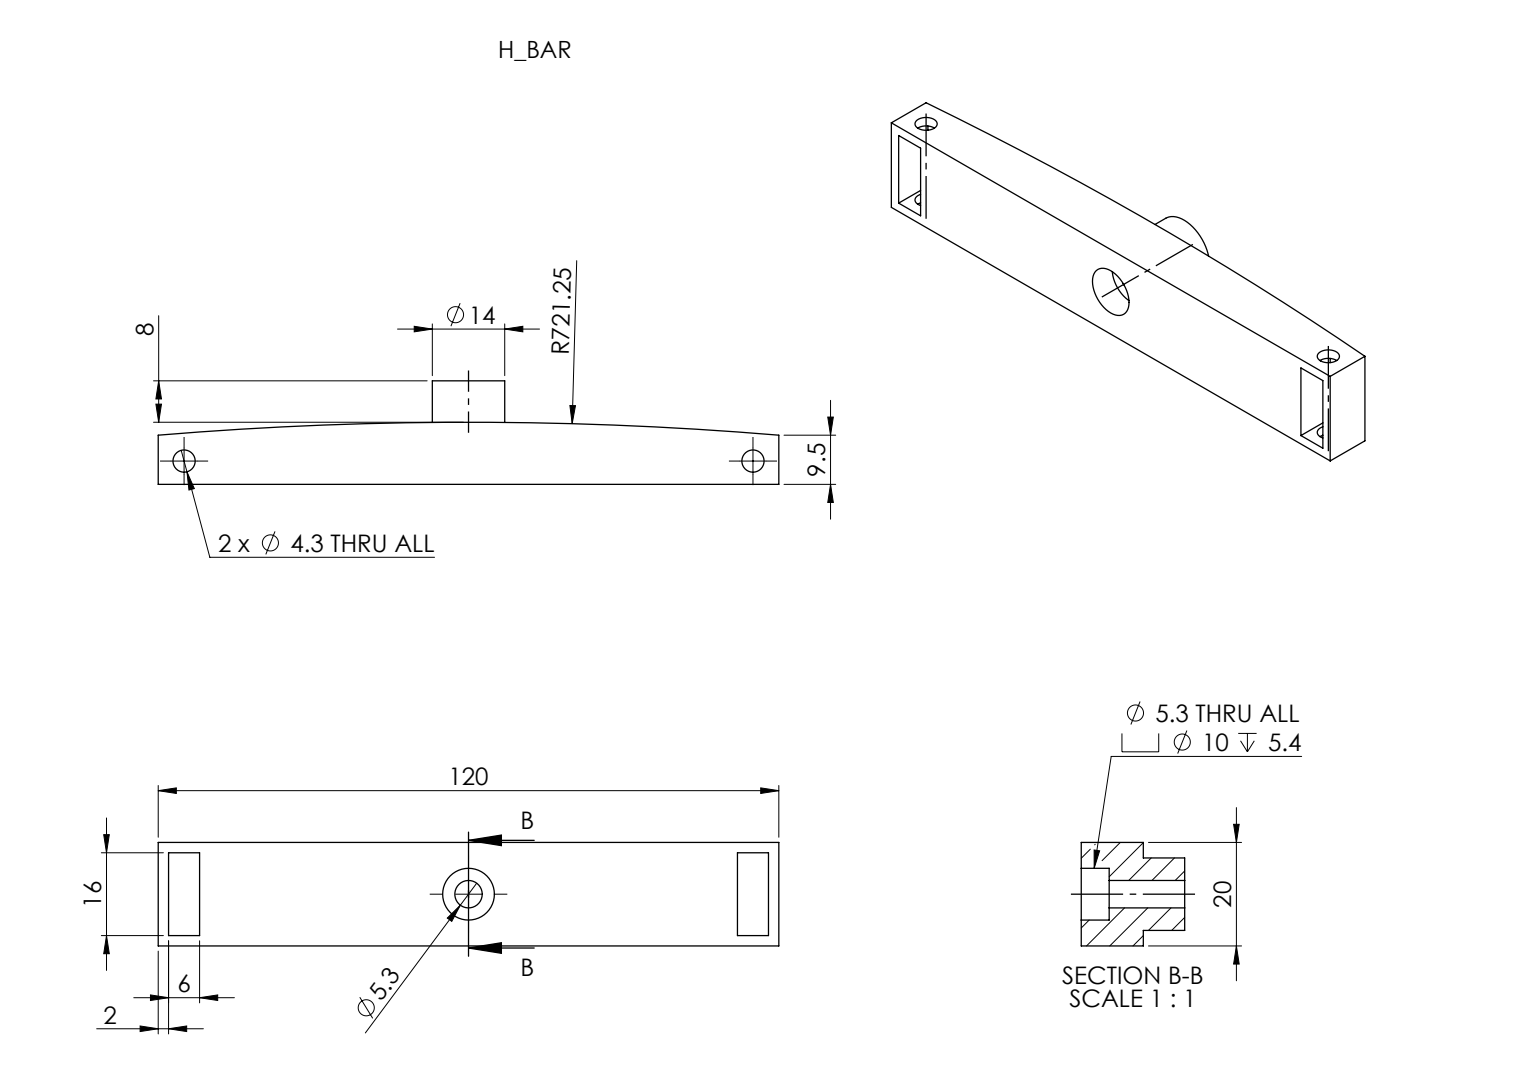
ISO-10303-21;
HEADER;
FILE_DESCRIPTION (('STEP AP214'),
    '1' );
FILE_NAME ('H_bar.step',
    '2026-10-08T12:12:07',
    ( '' ),
    ( '' ),
    'SwSTEP 2.0',
    'SolidWorks 2026',
    '' );
FILE_SCHEMA (( 'AUTOMOTIVE_DESIGN' ));
ENDSEC;

DATA;
#33=EDGE_CURVE ( 'NONE', #5370, #4266, #4037, .T. ) ;
#35=DIRECTION ( 'NONE',  ( 0.000000000000000000, -0.000000000000000000, -1.000000000000000000 ) ) ;
#36=CARTESIAN_POINT ( 'NONE',  ( -54.99999999999990052, 7.999999999999996447, 17.64999999999876579 ) ) ;
#37=CARTESIAN_POINT ( 'NONE',  ( 2.649999999999999023, 0.000000000000000000, 20.00000000000000355 ) ) ;
#43=ORIENTED_EDGE ( 'NONE', *, *, #111, .F. ) ;
#49=ORIENTED_EDGE ( 'NONE', *, *, #6995, .T. ) ;
#50=EDGE_CURVE ( 'NONE', #5044, #7574, #6013, .T. ) ;
#62=FACE_OUTER_BOUND ( 'NONE', #6300, .T. ) ;
#67=FACE_OUTER_BOUND ( 'NONE', #4002, .T. ) ;
#88=EDGE_CURVE ( 'NONE', #1891, #7622, #3368, .T. ) ;
#95=DIRECTION ( 'NONE',  ( -1.000000000000000000, 0.000000000000000000, 7.304098846218136639E-16 ) ) ;
#98=FACE_OUTER_BOUND ( 'NONE', #4834, .T. ) ;
#99=VECTOR ( 'NONE', #2043, 1000.000000000000000 ) ;
#103=CARTESIAN_POINT ( 'NONE',  ( 57.99999999999999289, 7.999999999999996447, 11.99999999999998934 ) ) ;
#111=EDGE_CURVE ( 'NONE', #2701, #7610, #4070, .T. ) ;
#120=VECTOR ( 'NONE', #1322, 1000.000000000000000 ) ;
#125=DIRECTION ( 'NONE',  ( 0.000000000000000000, 0.000000000000000000, 1.000000000000000000 ) ) ;
#130=AXIS2_PLACEMENT_3D ( 'NONE', #7551, #5648, #7466 ) ;
#132=ORIENTED_EDGE ( 'NONE', *, *, #3473, .T. ) ;
#142=CARTESIAN_POINT ( 'NONE',  ( 60.00000000000000711, 10.00000000000000000, 19.99999999999998224 ) ) ;
#147=EDGE_CURVE ( 'NONE', #4940, #6473, #5403, .T. ) ;
#149=ORIENTED_EDGE ( 'NONE', *, *, #1842, .T. ) ;
#156=CIRCLE ( 'NONE', #5095, 721.2499999999977263 ) ;
#162=ORIENTED_EDGE ( 'NONE', *, *, #3354, .T. ) ;
#179=EDGE_CURVE ( 'NONE', #2593, #4900, #5449, .T. ) ;
#188=LINE ( 'NONE', #4647, #2150 ) ;
#193=CARTESIAN_POINT ( 'NONE',  ( 52.00000000000000000, 7.999999999999996447, 19.99999999999998934 ) ) ;
#203=CARTESIAN_POINT ( 'NONE',  ( 1.817638007539982281, -6.775366854781982084, 8.002150721412645495 ) ) ;
#239=CIRCLE ( 'NONE', #4755, 2.650000000000010125 ) ;
#240=ORIENTED_EDGE ( 'NONE', *, *, #3379, .F. ) ;
#247=CARTESIAN_POINT ( 'NONE',  ( 6.063862694340463655, -3.504607373393594294, 8.025483085394268912 ) ) ;
#249=AXIS2_PLACEMENT_3D ( 'NONE', #6671, #347, #6580 ) ;
#253=EDGE_CURVE ( 'NONE', #6951, #2122, #5644, .T. ) ;
#262=DIRECTION ( 'NONE',  ( 0.000000000000000000, 0.000000000000000000, -1.000000000000000000 ) ) ;
#284=ORIENTED_EDGE ( 'NONE', *, *, #776, .T. ) ;
#286=CARTESIAN_POINT ( 'NONE',  ( 6.775412730438223896, -1.817364742217071338, 8.031819226609355766 ) ) ;
#289=PRODUCT_DEFINITION_FORMATION_WITH_SPECIFIED_SOURCE ( 'ANY', '', #1201, .NOT_KNOWN. ) ;
#292=EDGE_CURVE ( 'NONE', #5760, #2794, #1287, .T. ) ;
#313=CIRCLE ( 'NONE', #3509, 7.000000000000000000 ) ;
#315=EDGE_LOOP ( 'NONE', ( #5277, #4331 ) ) ;
#323=ORIENTED_EDGE ( 'NONE', *, *, #6415, .F. ) ;
#329=EDGE_CURVE ( 'NONE', #4266, #3008, #313, .T. ) ;
#335=SURFACE_STYLE_USAGE ( .BOTH. , #876 ) ;
#337=CARTESIAN_POINT ( 'NONE',  ( 55.00000000000000000, -8.000000000000001776, 17.64999999999999858 ) ) ;
#347=DIRECTION ( 'NONE',  ( -0.000000000000000000, 1.000000000000000000, -0.000000000000000000 ) ) ;
#350=LINE ( 'NONE', #2279, #863 ) ;
#357=DIRECTION ( 'NONE',  ( 0.000000000000000000, 0.000000000000000000, 1.000000000000000000 ) ) ;
#361=CARTESIAN_POINT ( 'NONE',  ( -58.00000000000006395, -8.000000000000003553, 19.99999999999998934 ) ) ;
#364=EDGE_LOOP ( 'NONE', ( #6417, #7648 ) ) ;
#369=CARTESIAN_POINT ( 'NONE',  ( -60.00000000000000000, 10.00000000000000000, 20.00000000000000355 ) ) ;
#370=CARTESIAN_POINT ( 'NONE',  ( -3.469446951953613006E-15, 0.000000000000000000, 20.00000000000000355 ) ) ;
#382=CARTESIAN_POINT ( 'NONE',  ( -6.821151181492251858, -1.588688383954758754, 8.032254533892484005 ) ) ;
#385=DIRECTION ( 'NONE',  ( -1.000000000000000000, 0.000000000000000000, -0.000000000000000000 ) ) ;
#398=EDGE_CURVE ( 'NONE', #2960, #580, #3789, .T. ) ;
#399=CARTESIAN_POINT ( 'NONE',  ( -3.469446951953613006E-15, 0.000000000000000000, 14.60000000000000142 ) ) ;
#400=EDGE_CURVE ( 'NONE', #3913, #5044, #2617, .T. ) ;
#417=VECTOR ( 'NONE', #2244, 1000.000000000000000 ) ;
#426=CARTESIAN_POINT ( 'NONE',  ( -7.000000000000002665, -0.4626139278909737751, 8.033969604113735841 ) ) ;
#427=CARTESIAN_POINT ( 'NONE',  ( 5.563937487951679195, 4.272621587589405578, 8.021415735625629040 ) ) ;
#431=FILL_AREA_STYLE ('',( #5077 ) ) ;
#439=CARTESIAN_POINT ( 'NONE',  ( 52.00000000000000000, 7.999999999999996447, 19.99999999999998934 ) ) ;
#454=ADVANCED_FACE ( 'NONE', ( #5886, #6459 ), #5961, .F. ) ;
#458=CYLINDRICAL_SURFACE ( 'NONE', #3417, 4.999999999999993783 ) ;
#466=DIRECTION ( 'NONE',  ( 0.000000000000000000, -1.000000000000000000, 0.000000000000000000 ) ) ;
#470=CARTESIAN_POINT ( 'NONE',  ( 4.263933714126141972, 5.556256305342602175, 8.012582018583044530 ) ) ;
#471=VERTEX_POINT ( 'NONE', #2181 ) ;
#481=CARTESIAN_POINT ( 'NONE',  ( 9.020562075079396891E-14, 10.00000000000000000, 8.000000000000007105 ) ) ;
#485=EDGE_CURVE ( 'NONE', #5247, #2461, #7128, .T. ) ;
#492=ORIENTED_EDGE ( 'NONE', *, *, #3666, .F. ) ;
#496=DIRECTION ( 'NONE',  ( -0.000000000000000000, 1.000000000000000000, -0.000000000000000000 ) ) ;
#497=CARTESIAN_POINT ( 'NONE',  ( -58.00000000000006395, -8.000000000000003553, 11.99999999999998934 ) ) ;
#503=DIRECTION ( 'NONE',  ( -0.000000000000000000, -0.000000000000000000, 1.000000000000000000 ) ) ;
#533=ORIENTED_EDGE ( 'NONE', *, *, #8046, .T. ) ;
#537=DIRECTION ( 'NONE',  ( 0.000000000000000000, -1.000000000000000000, 0.000000000000000000 ) ) ;
#542=CIRCLE ( 'NONE', #6772, 2.149999999999995470 ) ;
#545=EDGE_LOOP ( 'NONE', ( #3135, #132, #1061, #2329, #6550 ) ) ;
#562=AXIS2_PLACEMENT_3D ( 'NONE', #5807, #845, #6662 ) ;
#579=EDGE_LOOP ( 'NONE', ( #6634, #3876, #4463, #3342 ) ) ;
#580=VERTEX_POINT ( 'NONE', #4679 ) ;
#585=FACE_OUTER_BOUND ( 'NONE', #4794, .T. ) ;
#615=LINE ( 'NONE', #8136, #2509 ) ;
#622=ORIENTED_EDGE ( 'NONE', *, *, #7733, .F. ) ;
#625=ORIENTED_EDGE ( 'NONE', *, *, #147, .F. ) ;
#627=CARTESIAN_POINT ( 'NONE',  ( -52.00000000000006395, 7.999999999999996447, 19.99999999999998934 ) ) ;
#628=CARTESIAN_POINT ( 'NONE',  ( -3.469446951953613006E-15, 0.000000000000000000, 1.040834085586084257E-14 ) ) ;
#630=ORIENTED_EDGE ( 'NONE', *, *, #4013, .F. ) ;
#639=CARTESIAN_POINT ( 'NONE',  ( -3.469446951953613006E-15, 0.000000000000000000, 20.00000000000000355 ) ) ;
#660=DIRECTION ( 'NONE',  ( -0.000000000000000000, 1.000000000000000000, -0.000000000000000000 ) ) ;
#661=VECTOR ( 'NONE', #6389, 1000.000000000000000 ) ;
#664=CARTESIAN_POINT ( 'NONE',  ( -54.99999999999990052, 10.00000000000000000, 13.34999999999877218 ) ) ;
#674=ORIENTED_EDGE ( 'NONE', *, *, #5759, .F. ) ;
#692=PLANE ( 'NONE',  #3596 ) ;
#698=CARTESIAN_POINT ( 'NONE',  ( -2.649999999999998579, 3.245314017740484976E-16, 1.040834085586084257E-14 ) ) ;
#710=DIRECTION ( 'NONE',  ( 0.000000000000000000, 0.000000000000000000, -1.000000000000000000 ) ) ;
#718=EDGE_CURVE ( 'NONE', #6876, #5247, #3796, .T. ) ;
#725=EDGE_CURVE ( 'NONE', #4369, #7382, #3169, .T. ) ;
#729=FACE_OUTER_BOUND ( 'NONE', #7926, .T. ) ;
#736=ORIENTED_EDGE ( 'NONE', *, *, #147, .T. ) ;
#737=ORIENTED_EDGE ( 'NONE', *, *, #4756, .F. ) ;
#745=CARTESIAN_POINT ( 'NONE',  ( -54.99999999999990052, 7.999999999999996447, 15.49999999999877254 ) ) ;
#746=ORIENTED_EDGE ( 'NONE', *, *, #292, .T. ) ;
#747=ORIENTED_EDGE ( 'NONE', *, *, #7686, .F. ) ;
#751=DIRECTION ( 'NONE',  ( -0.000000000000000000, 1.000000000000000000, -0.000000000000000000 ) ) ;
#755=AXIS2_PLACEMENT_3D ( 'NONE', #7446, #2992, #997 ) ;
#756=CIRCLE ( 'NONE', #6069, 2.149999999999995470 ) ;
#759=DIRECTION ( 'NONE',  ( 0.000000000000000000, 0.000000000000000000, 1.000000000000000000 ) ) ;
#762=LINE ( 'NONE', #7672, #2341 ) ;
#764=ORIENTED_EDGE ( 'NONE', *, *, #3354, .F. ) ;
#765=DIRECTION ( 'NONE',  ( -0.000000000000000000, -0.000000000000000000, 1.000000000000000000 ) ) ;
#769=FACE_BOUND ( 'NONE', #5362, .T. ) ;
#775=VECTOR ( 'NONE', #2784, 1000.000000000000000 ) ;
#776=EDGE_CURVE ( 'NONE', #7532, #6647, #3721, .T. ) ;
#783=EDGE_LOOP ( 'NONE', ( #2328, #2669, #3779, #4427 ) ) ;
#796=CARTESIAN_POINT ( 'NONE',  ( -58.00000000000006395, -8.000000000000003553, 11.99999999999998934 ) ) ;
#797=EDGE_CURVE ( 'NONE', #3149, #2513, #8163, .T. ) ;
#805=CARTESIAN_POINT ( 'NONE',  ( 60.00000000000000711, 10.00000000000000000, 19.99999999999998224 ) ) ;
#812=LINE ( 'NONE', #1377, #1681 ) ;
#813=LINE ( 'NONE', #4683, #1169 ) ;
#816=CARTESIAN_POINT ( 'NONE',  ( 9.020562075079396891E-14, 10.00000000000000000, 729.2499999999977263 ) ) ;
#831=CARTESIAN_POINT ( 'NONE',  ( -3.469446951953613006E-15, 0.000000000000000000, 20.00000000000000355 ) ) ;
#833=( GEOMETRIC_REPRESENTATION_CONTEXT ( 3 ) GLOBAL_UNCERTAINTY_ASSIGNED_CONTEXT ( ( #1043 ) ) GLOBAL_UNIT_ASSIGNED_CONTEXT ( ( #7363, #5472, #1683 ) ) REPRESENTATION_CONTEXT ( 'NONE', 'WORKASPACE' ) );
#835=CARTESIAN_POINT ( 'NONE',  ( 60.00000000000000711, 10.00000000000000000, 19.99999999999998224 ) ) ;
#836=ADVANCED_FACE ( 'NONE', ( #2976 ), #4986, .T. ) ;
#838=EDGE_CURVE ( 'NONE', #5760, #2420, #5577, .T. ) ;
#841=DIRECTION ( 'NONE',  ( 0.000000000000000000, 0.000000000000000000, 1.000000000000000000 ) ) ;
#845=DIRECTION ( 'NONE',  ( -0.000000000000000000, -0.000000000000000000, 1.000000000000000000 ) ) ;
#863=VECTOR ( 'NONE', #7874, 1000.000000000000000 ) ;
#864=ORIENTED_EDGE ( 'NONE', *, *, #4147, .T. ) ;
#865=DIRECTION ( 'NONE',  ( 0.000000000000000000, -1.000000000000000000, 0.000000000000000000 ) ) ;
#870=AXIS2_PLACEMENT_3D ( 'NONE', #103, #5737, #2689 ) ;
#873=DIRECTION ( 'NONE',  ( 0.000000000000000000, 0.000000000000000000, 1.000000000000000000 ) ) ;
#875=B_SPLINE_CURVE_WITH_KNOTS ( 'NONE', 3,
 ( #6650, #6025, #2207, #203, #2749, #5292, #3377, #4666, #2168, #2092, #7318, #914, #2714, #5986, #247, #3500, #4704, #2797, #286, #4791, #957, #4623 ),
 .UNSPECIFIED., .F., .F.,
 ( 4, 2, 2, 2, 2, 2, 2, 2, 2, 2, 4 ),
 ( 0.01094514227676123691, 0.01231266565124741405, 0.01368018902573359119, 0.01436395071297667803, 0.01504771240021976486, 0.01641523577470593853, 0.01778275914919211220, 0.01846652083643519904, 0.01915028252367827893, 0.02051780589816445260, 0.02188532927265061934 ),
 .UNSPECIFIED. ) ;
#876=SURFACE_SIDE_STYLE ('',( #6615 ) ) ;
#882=EDGE_LOOP ( 'NONE', ( #6137, #7790, #7495, #985 ) ) ;
#885=DIRECTION ( 'NONE',  ( 0.000000000000000000, 0.000000000000000000, -1.000000000000000000 ) ) ;
#895=EDGE_LOOP ( 'NONE', ( #149, #7973 ) ) ;
#908=ORIENTED_EDGE ( 'NONE', *, *, #1318, .T. ) ;
#914=CARTESIAN_POINT ( 'NONE',  ( 5.276116561136752203, -4.623420808406671689, 8.019224293709841689 ) ) ;
#923=CARTESIAN_POINT ( 'NONE',  ( 55.00000000000000000, 7.999999999999996447, 15.50000000000000355 ) ) ;
#927=APPLICATION_CONTEXT ( 'automotive_design' ) ;
#929=DIRECTION ( 'NONE',  ( 1.000000000000000000, 0.000000000000000000, -1.734723475976807094E-16 ) ) ;
#938=CARTESIAN_POINT ( 'NONE',  ( 57.99999999999999289, 7.999999999999996447, 11.99999999999998934 ) ) ;
#943=ORIENTED_EDGE ( 'NONE', *, *, #5994, .T. ) ;
#945=EDGE_CURVE ( 'NONE', #2445, #7873, #4769, .T. ) ;
#947=CARTESIAN_POINT ( 'NONE',  ( -54.99999999999990052, -8.000000000000001776, 13.34999999999877573 ) ) ;
#957=CARTESIAN_POINT ( 'NONE',  ( 7.000000000000000000, -0.4567577452614210998, 8.033969604113657681 ) ) ;
#963=ADVANCED_FACE ( 'NONE', ( #4403 ), #7637, .F. ) ;
#967=PLANE ( 'NONE',  #3326 ) ;
#980=LINE ( 'NONE', #938, #4549 ) ;
#984=ORIENTED_EDGE ( 'NONE', *, *, #6326, .T. ) ;
#985=ORIENTED_EDGE ( 'NONE', *, *, #7008, .T. ) ;
#988=CARTESIAN_POINT ( 'NONE',  ( 55.00000000000000000, 7.999999999999996447, 17.64999999999999858 ) ) ;
#997=DIRECTION ( 'NONE',  ( 0.000000000000000000, 0.000000000000000000, -1.000000000000000000 ) ) ;
#999=ORIENTED_EDGE ( 'NONE', *, *, #1723, .T. ) ;
#1007=CIRCLE ( 'NONE', #3821, 2.149999999999992362 ) ;
#1008=ADVANCED_FACE ( 'NONE', ( #3156, #7748 ), #692, .F. ) ;
#1009=EDGE_CURVE ( 'NONE', #2513, #7631, #542, .T. ) ;
#1011=FACE_OUTER_BOUND ( 'NONE', #3128, .T. ) ;
#1012=ORIENTED_EDGE ( 'NONE', *, *, #945, .F. ) ;
#1020=ORIENTED_EDGE ( 'NONE', *, *, #4149, .F. ) ;
#1022=ORIENTED_EDGE ( 'NONE', *, *, #3595, .F. ) ;
#1032=AXIS2_PLACEMENT_3D ( 'NONE', #745, #2051, #5285 ) ;
#1039=CARTESIAN_POINT ( 'NONE',  ( 0.000000000000000000, 0.000000000000000000, 0.000000000000000000 ) ) ;
#1043=UNCERTAINTY_MEASURE_WITH_UNIT (LENGTH_MEASURE( 1.000000000000000082E-05 ), #7363, 'distance_accuracy_value', 'NONE');
#1057=FACE_OUTER_BOUND ( 'NONE', #7251, .T. ) ;
#1059=ORIENTED_EDGE ( 'NONE', *, *, #7565, .F. ) ;
#1061=ORIENTED_EDGE ( 'NONE', *, *, #2412, .T. ) ;
#1068=EDGE_LOOP ( 'NONE', ( #6038, #2674, #6851, #8178 ) ) ;
#1071=ORIENTED_EDGE ( 'NONE', *, *, #8119, .F. ) ;
#1083=CARTESIAN_POINT ( 'NONE',  ( -60.00000000000000000, -10.00000000000000000, 10.50000000000000000 ) ) ;
#1091=DIRECTION ( 'NONE',  ( -0.000000000000000000, 1.000000000000000000, -0.000000000000000000 ) ) ;
#1101=EDGE_LOOP ( 'NONE', ( #4231, #1354, #3513, #6258 ) ) ;
#1107=DIRECTION ( 'NONE',  ( 0.000000000000000000, 1.000000000000000000, -0.000000000000000000 ) ) ;
#1116=CARTESIAN_POINT ( 'NONE',  ( -1.809537700406288696, 6.765955536481263799, 8.002236580937831079 ) ) ;
#1127=LINE ( 'NONE', #6150, #6601 ) ;
#1131=CYLINDRICAL_SURFACE ( 'NONE', #4595, 4.999999999999993783 ) ;
#1152=PLANE ( 'NONE',  #2816 ) ;
#1169=VECTOR ( 'NONE', #6434, 1000.000000000000000 ) ;
#1175=CIRCLE ( 'NONE', #5826, 2.649999999999995026 ) ;
#1189=EDGE_LOOP ( 'NONE', ( #4336, #622, #5682, #3680 ) ) ;
#1197=VECTOR ( 'NONE', #3237, 1000.000000000000000 ) ;
#1201=PRODUCT ( 'H_bar', 'H_bar', '', ( #3408 ) ) ;
#1205=CARTESIAN_POINT ( 'NONE',  ( 55.00000000000000000, -8.000000000000001776, 13.35000000000000853 ) ) ;
#1209=LINE ( 'NONE', #37, #3965 ) ;
#1242=CARTESIAN_POINT ( 'NONE',  ( -54.99999999999990052, -8.000000000000001776, 15.49999999999877254 ) ) ;
#1275=ORIENTED_EDGE ( 'NONE', *, *, #838, .F. ) ;
#1280=CARTESIAN_POINT ( 'NONE',  ( -60.00000000000000000, -10.00000000000000000, 20.00000000000000355 ) ) ;
#1282=EDGE_CURVE ( 'NONE', #5386, #4369, #4820, .T. ) ;
#1287=LINE ( 'NONE', #5085, #2062 ) ;
#1307=ORIENTED_EDGE ( 'NONE', *, *, #1889, .T. ) ;
#1308=ORIENTED_EDGE ( 'NONE', *, *, #400, .T. ) ;
#1313=CARTESIAN_POINT ( 'NONE',  ( -0.4566803630309465567, -7.000000000000006217, 8.000000000000042633 ) ) ;
#1315=ADVANCED_FACE ( 'NONE', ( #4557 ), #3144, .T. ) ;
#1318=EDGE_CURVE ( 'NONE', #6647, #5567, #5729, .T. ) ;
#1320=DIRECTION ( 'NONE',  ( -0.000000000000000000, 1.000000000000000000, -0.000000000000000000 ) ) ;
#1322=DIRECTION ( 'NONE',  ( -7.304098846218136639E-16, 0.000000000000000000, -1.000000000000000000 ) ) ;
#1331=ORIENTED_EDGE ( 'NONE', *, *, #179, .T. ) ;
#1337=CARTESIAN_POINT ( 'NONE',  ( 9.020562075079396891E-14, 10.00000000000000000, 729.2499999999977263 ) ) ;
#1342=VECTOR ( 'NONE', #7696, 1000.000000000000000 ) ;
#1354=ORIENTED_EDGE ( 'NONE', *, *, #3875, .F. ) ;
#1361=DIRECTION ( 'NONE',  ( -0.000000000000000000, -0.000000000000000000, 1.000000000000000000 ) ) ;
#1368=SHAPE_REPRESENTATION ( 'H_bar', ( #1587 ), #2170 ) ;
#1377=CARTESIAN_POINT ( 'NONE',  ( 52.00000000000000000, 7.999999999999996447, 11.99999999999998934 ) ) ;
#1381=ORIENTED_EDGE ( 'NONE', *, *, #725, .F. ) ;
#1389=CARTESIAN_POINT ( 'NONE',  ( -54.99999999999990052, -8.000000000000001776, 17.64999999999876579 ) ) ;
#1393=ORIENTED_EDGE ( 'NONE', *, *, #6516, .T. ) ;
#1399=CARTESIAN_POINT ( 'NONE',  ( -3.094755790304997145, -6.282913975126477979, 8.006611220574070487 ) ) ;
#1400=VECTOR ( 'NONE', #765, 1000.000000000000000 ) ;
#1421=AXIS2_PLACEMENT_3D ( 'NONE', #4138, #4718, #1488 ) ;
#1423=CARTESIAN_POINT ( 'NONE',  ( 52.00000000000000000, -8.000000000000003553, 11.99999999999998934 ) ) ;
#1430=EDGE_LOOP ( 'NONE', ( #2699, #674, #6368, #3754 ) ) ;
#1445=DIRECTION ( 'NONE',  ( -0.000000000000000000, 1.000000000000000000, -0.000000000000000000 ) ) ;
#1448=CARTESIAN_POINT ( 'NONE',  ( 2.650000000000006573, 0.000000000000000000, 14.60000000000000142 ) ) ;
#1461=VERTEX_POINT ( 'NONE', #835 ) ;
#1482=CYLINDRICAL_SURFACE ( 'NONE', #7579, 2.149999999999995470 ) ;
#1488=DIRECTION ( 'NONE',  ( -1.000000000000000000, 0.000000000000000000, 0.000000000000000000 ) ) ;
#1503=ORIENTED_EDGE ( 'NONE', *, *, #4756, .T. ) ;
#1516=( NAMED_UNIT ( * ) SI_UNIT ( $, .STERADIAN. ) SOLID_ANGLE_UNIT ( ) );
#1518=CARTESIAN_POINT ( 'NONE',  ( 6.764948177723724143, 1.813303243961031264, 8.031723462610594666 ) ) ;
#1544=FACE_BOUND ( 'NONE', #3563, .T. ) ;
#1551=FILL_AREA_STYLE ('',( #6745 ) ) ;
#1557=STYLED_ITEM ( 'NONE', ( #1912 ), #6918 ) ;
#1562=DIRECTION ( 'NONE',  ( -7.304098846218136639E-16, 0.000000000000000000, -1.000000000000000000 ) ) ;
#1565=CARTESIAN_POINT ( 'NONE',  ( 55.00000000000000000, 10.00000000000000000, 17.65000000000000213 ) ) ;
#1581=CARTESIAN_POINT ( 'NONE',  ( -5.560873836092222078, 4.276402017733387240, 8.021392354376160938 ) ) ;
#1585=ADVANCED_FACE ( 'NONE', ( #4332 ), #1131, .F. ) ;
#1587=AXIS2_PLACEMENT_3D ( 'NONE', #3942, #5152, #6454 ) ;
#1588=ORIENTED_EDGE ( 'NONE', *, *, #3229, .F. ) ;
#1611=LINE ( 'NONE', #2935, #3551 ) ;
#1612=CARTESIAN_POINT ( 'NONE',  ( 55.00000000000000000, 7.999999999999996447, 13.35000000000000853 ) ) ;
#1613=LINE ( 'NONE', #7372, #4745 ) ;
#1615=CARTESIAN_POINT ( 'NONE',  ( -52.00000000000006395, -8.000000000000003553, 11.99999999999998934 ) ) ;
#1625=CARTESIAN_POINT ( 'NONE',  ( -7.000000000000000000, 0.4621588634683668206, 8.033969604113732288 ) ) ;
#1628=AXIS2_PLACEMENT_3D ( 'NONE', #2103, #4640, #7863 ) ;
#1638=DIRECTION ( 'NONE',  ( -0.000000000000000000, -1.000000000000000000, -0.000000000000000000 ) ) ;
#1642=MECHANICAL_DESIGN_GEOMETRIC_PRESENTATION_REPRESENTATION('',(#5233),#833);
#1644=DIRECTION ( 'NONE',  ( -0.000000000000000000, 1.000000000000000000, -0.000000000000000000 ) ) ;
#1645=CARTESIAN_POINT ( 'NONE',  ( -6.290416253262643309, -3.105047250628316213, 8.027410178832276699 ) ) ;
#1657=EDGE_LOOP ( 'NONE', ( #1071, #737 ) ) ;
#1660=ORIENTED_EDGE ( 'NONE', *, *, #5235, .T. ) ;
#1669=ORIENTED_EDGE ( 'NONE', *, *, #3413, .F. ) ;
#1681=VECTOR ( 'NONE', #5239, 1000.000000000000000 ) ;
#1682=AXIS2_PLACEMENT_3D ( 'NONE', #4853, #2353, #4946 ) ;
#1683=( NAMED_UNIT ( * ) SI_UNIT ( $, .STERADIAN. ) SOLID_ANGLE_UNIT ( ) );
#1685=CARTESIAN_POINT ( 'NONE',  ( 6.282784822387311507, 3.095002094042488050, 8.027357021320174368 ) ) ;
#1690=DIRECTION ( 'NONE',  ( -0.000000000000000000, -1.000000000000000000, -0.000000000000000000 ) ) ;
#1700=VECTOR ( 'NONE', #5315, 1000.000000000000000 ) ;
#1723=EDGE_CURVE ( 'NONE', #7610, #1891, #350, .T. ) ;
#1727=VERTEX_POINT ( 'NONE', #2899 ) ;
#1743=DIRECTION ( 'NONE',  ( 1.000000000000000000, 0.000000000000000000, -1.734723475976807094E-16 ) ) ;
#1748=ORIENTED_EDGE ( 'NONE', *, *, #3669, .T. ) ;
#1749=ORIENTED_EDGE ( 'NONE', *, *, #2036, .T. ) ;
#1759=ORIENTED_EDGE ( 'NONE', *, *, #8046, .F. ) ;
#1765=CIRCLE ( 'NONE', #3887, 4.999999999999993783 ) ;
#1771=CARTESIAN_POINT ( 'NONE',  ( -54.99999999999990052, 10.00000000000000000, 15.49999999999877254 ) ) ;
#1774=CARTESIAN_POINT ( 'NONE',  ( 9.020562070449730010E-14, 7.000000000000000000, 8.000000000000058620 ) ) ;
#1780=DIRECTION ( 'NONE',  ( 0.000000000000000000, 1.000000000000000000, -0.000000000000000000 ) ) ;
#1787=ORIENTED_EDGE ( 'NONE', *, *, #2211, .F. ) ;
#1813=CARTESIAN_POINT ( 'NONE',  ( -3.469446951953613006E-15, 0.000000000000000000, 14.60000000000000142 ) ) ;
#1815=CARTESIAN_POINT ( 'NONE',  ( -54.99999999999990052, -10.00000000000000000, 13.34999999999877929 ) ) ;
#1817=CARTESIAN_POINT ( 'NONE',  ( 2.468988737128785083, 6.554131952896964819, 8.004194855151794741 ) ) ;
#1832=CARTESIAN_POINT ( 'NONE',  ( -3.469446951953613006E-15, 0.000000000000000000, 14.60000000000000142 ) ) ;
#1839=AXIS2_PLACEMENT_3D ( 'NONE', #3556, #4717, #885 ) ;
#1842=EDGE_CURVE ( 'NONE', #4940, #5103, #3404, .T. ) ;
#1846=EDGE_CURVE ( 'NONE', #5782, #2794, #8037, .T. ) ;
#1863=DIRECTION ( 'NONE',  ( 1.000000000000000000, 0.000000000000000000, 0.000000000000000000 ) ) ;
#1865=CARTESIAN_POINT ( 'NONE',  ( 3.506487216771620563, 6.075720677264023095, 8.008423154362855456 ) ) ;
#1880=CARTESIAN_POINT ( 'NONE',  ( -58.00000000000006395, -8.000000000000003553, 19.99999999999998934 ) ) ;
#1889=EDGE_CURVE ( 'NONE', #2122, #6951, #1007, .T. ) ;
#1891=VERTEX_POINT ( 'NONE', #439 ) ;
#1896=ORIENTED_EDGE ( 'NONE', *, *, #1842, .F. ) ;
#1905=DIRECTION ( 'NONE',  ( 0.000000000000000000, -1.000000000000000000, 0.000000000000000000 ) ) ;
#1912=PRESENTATION_STYLE_ASSIGNMENT (( #4890 ) ) ;
#1915=FACE_OUTER_BOUND ( 'NONE', #1189, .T. ) ;
#1932=ORIENTED_EDGE ( 'NONE', *, *, #33, .T. ) ;
#1942=ORIENTED_EDGE ( 'NONE', *, *, #4581, .T. ) ;
#1945=DIRECTION ( 'NONE',  ( -0.000000000000000000, -0.000000000000000000, 1.000000000000000000 ) ) ;
#1949=CYLINDRICAL_SURFACE ( 'NONE', #7815, 2.149999999999995470 ) ;
#1958=ORIENTED_EDGE ( 'NONE', *, *, #6729, .T. ) ;
#1982=DIRECTION ( 'NONE',  ( 0.000000000000000000, -1.000000000000000000, 0.000000000000000000 ) ) ;
#1986=CARTESIAN_POINT ( 'NONE',  ( -0.9110278382907691652, -6.955741332015764833, 8.000433768563103953 ) ) ;
#1988=VECTOR ( 'NONE', #4498, 1000.000000000000000 ) ;
#1993=DIRECTION ( 'NONE',  ( 1.000000000000000000, 0.000000000000000000, 0.000000000000000000 ) ) ;
#1999=ADVANCED_FACE ( 'NONE', ( #5997, #7749 ), #2614, .F. ) ;
#2006=PLANE ( 'NONE',  #4510 ) ;
#2009=ORIENTED_EDGE ( 'NONE', *, *, #1846, .T. ) ;
#2010=AXIS2_PLACEMENT_3D ( 'NONE', #2629, #4499, #3883 ) ;
#2011=ORIENTED_EDGE ( 'NONE', *, *, #4937, .T. ) ;
#2028=CARTESIAN_POINT ( 'NONE',  ( -4.624865572637439470, -5.274399087326279378, 8.014755761910349108 ) ) ;
#2030=CARTESIAN_POINT ( 'NONE',  ( 55.00000000000000000, 10.00000000000000000, 15.50000000000000355 ) ) ;
#2036=EDGE_CURVE ( 'NONE', #5534, #1891, #762, .T. ) ;
#2042=ADVANCED_FACE ( 'NONE', ( #62 ), #5772, .F. ) ;
#2043=DIRECTION ( 'NONE',  ( -0.000000000000000000, 1.000000000000000000, -0.000000000000000000 ) ) ;
#2050=CARTESIAN_POINT ( 'NONE',  ( -2.650000000000013678, 3.245314017740498288E-16, 14.60000000000000142 ) ) ;
#2051=DIRECTION ( 'NONE',  ( 0.000000000000000000, 1.000000000000000000, -0.000000000000000000 ) ) ;
#2062=VECTOR ( 'NONE', #660, 1000.000000000000000 ) ;
#2068=ORIENTED_EDGE ( 'NONE', *, *, #6931, .T. ) ;
#2073=ADVANCED_FACE ( 'NONE', ( #729 ), #3274, .F. ) ;
#2092=CARTESIAN_POINT ( 'NONE',  ( 4.269299642044305010, -5.566066101761777851, 8.012536085362354399 ) ) ;
#2103=CARTESIAN_POINT ( 'NONE',  ( -54.99999999999990052, 10.00000000000000000, 15.49999999999877254 ) ) ;
#2122=VERTEX_POINT ( 'NONE', #5959 ) ;
#2133=DIRECTION ( 'NONE',  ( 0.000000000000000000, 0.000000000000000000, 1.000000000000000000 ) ) ;
#2148=DIRECTION ( 'NONE',  ( -1.000000000000000000, 0.000000000000000000, 0.000000000000000000 ) ) ;
#2150=VECTOR ( 'NONE', #7177, 1000.000000000000000 ) ;
#2151=ADVANCED_FACE ( 'NONE', ( #1011 ), #5884, .F. ) ;
#2153=ORIENTED_EDGE ( 'NONE', *, *, #6516, .F. ) ;
#2161=DIRECTION ( 'NONE',  ( 0.000000000000000000, -1.000000000000000000, 0.000000000000000000 ) ) ;
#2164=VERTEX_POINT ( 'NONE', #337 ) ;
#2168=CARTESIAN_POINT ( 'NONE',  ( 3.700545867704406966, -5.946256225702112097, 8.009468413176323409 ) ) ;
#2170=( GEOMETRIC_REPRESENTATION_CONTEXT ( 3 ) GLOBAL_UNCERTAINTY_ASSIGNED_CONTEXT ( ( #2378 ) ) GLOBAL_UNIT_ASSIGNED_CONTEXT ( ( #4089, #7825, #1516 ) ) REPRESENTATION_CONTEXT ( 'NONE', 'WORKASPACE' ) );
#2178=EDGE_CURVE ( 'NONE', #7471, #1461, #4094, .T. ) ;
#2181=CARTESIAN_POINT ( 'NONE',  ( 57.99999999999999289, -8.000000000000003553, 11.99999999999998934 ) ) ;
#2184=CARTESIAN_POINT ( 'NONE',  ( -7.000000000000000000, 0.000000000000000000, 0.000000000000000000 ) ) ;
#2190=ORIENTED_EDGE ( 'NONE', *, *, #945, .T. ) ;
#2199=LINE ( 'NONE', #7350, #2221 ) ;
#2207=CARTESIAN_POINT ( 'NONE',  ( 0.9200942725349188223, -6.954338967362795110, 8.000447262915827196 ) ) ;
#2211=EDGE_CURVE ( 'NONE', #5370, #4900, #6485, .T. ) ;
#2213=FACE_OUTER_BOUND ( 'NONE', #6917, .T. ) ;
#2219=ORIENTED_EDGE ( 'NONE', *, *, #2839, .F. ) ;
#2221=VECTOR ( 'NONE', #6724, 1000.000000000000000 ) ;
#2232=ADVANCED_FACE ( 'NONE', ( #4841, #3678, #1057, #8026 ), #3735, .F. ) ;
#2235=ORIENTED_EDGE ( 'NONE', *, *, #2412, .F. ) ;
#2244=DIRECTION ( 'NONE',  ( 0.000000000000000000, 0.000000000000000000, 1.000000000000000000 ) ) ;
#2257=FACE_OUTER_BOUND ( 'NONE', #4121, .T. ) ;
#2265=CARTESIAN_POINT ( 'NONE',  ( -7.000000000000000000, 1.843750452292770530E-16, 8.033969604113661234 ) ) ;
#2266=CARTESIAN_POINT ( 'NONE',  ( 6.955677005507068245, 0.9111895000360680230, 8.033535213607201797 ) ) ;
#2271=FACE_OUTER_BOUND ( 'NONE', #2307, .T. ) ;
#2279=CARTESIAN_POINT ( 'NONE',  ( 57.99999999999999289, 7.999999999999996447, 19.99999999999998934 ) ) ;
#2284=CARTESIAN_POINT ( 'NONE',  ( 55.00000000000000000, 10.00000000000000000, 15.50000000000000355 ) ) ;
#2287=CARTESIAN_POINT ( 'NONE',  ( -5.271309882437016370, 4.628374325350936402, 8.019190801808186109 ) ) ;
#2290=AXIS2_PLACEMENT_3D ( 'NONE', #7413, #5016, #385 ) ;
#2307=EDGE_LOOP ( 'NONE', ( #1787, #1932, #6522, #2866, #7072 ) ) ;
#2316=DIRECTION ( 'NONE',  ( 1.000000000000000000, 0.000000000000000000, 0.000000000000000000 ) ) ;
#2324=CARTESIAN_POINT ( 'NONE',  ( -4.999999999999997335, 6.123233995736758394E-16, 20.00000000000000355 ) ) ;
#2328=ORIENTED_EDGE ( 'NONE', *, *, #3057, .F. ) ;
#2329=ORIENTED_EDGE ( 'NONE', *, *, #5553, .T. ) ;
#2341=VECTOR ( 'NONE', #3320, 1000.000000000000000 ) ;
#2343=CARTESIAN_POINT ( 'NONE',  ( 1.587956359206372792, 6.821324887144850635, 8.001713349940533959 ) ) ;
#2347=( LENGTH_UNIT ( ) NAMED_UNIT ( * ) SI_UNIT ( .MILLI., .METRE. ) );
#2351=VECTOR ( 'NONE', #1638, 1000.000000000000000 ) ;
#2352=CARTESIAN_POINT ( 'NONE',  ( -54.99999999999990052, 7.999999999999996447, 15.49999999999877254 ) ) ;
#2353=DIRECTION ( 'NONE',  ( -0.000000000000000000, 1.000000000000000000, -0.000000000000000000 ) ) ;
#2357=DIRECTION ( 'NONE',  ( 0.000000000000000000, 0.000000000000000000, 1.000000000000000000 ) ) ;
#2359=DIRECTION ( 'NONE',  ( 0.000000000000000000, 0.000000000000000000, 1.000000000000000000 ) ) ;
#2366=CIRCLE ( 'NONE', #2901, 2.149999999999999023 ) ;
#2369=VECTOR ( 'NONE', #6804, 1000.000000000000000 ) ;
#2378=UNCERTAINTY_MEASURE_WITH_UNIT (LENGTH_MEASURE( 1.000000000000000082E-05 ), #4089, 'distance_accuracy_value', 'NONE');
#2385=EDGE_LOOP ( 'NONE', ( #6365, #764, #4734, #7342 ) ) ;
#2388=DIRECTION ( 'NONE',  ( 0.000000000000000000, 0.000000000000000000, 1.000000000000000000 ) ) ;
#2391=EDGE_CURVE ( 'NONE', #5793, #5534, #980, .T. ) ;
#2395=ORIENTED_EDGE ( 'NONE', *, *, #7434, .T. ) ;
#2398=SURFACE_SIDE_STYLE ('',( #7597 ) ) ;
#2399=LINE ( 'NONE', #4439, #6479 ) ;
#2412=EDGE_CURVE ( 'NONE', #2593, #6876, #156, .T. ) ;
#2417=EDGE_LOOP ( 'NONE', ( #284, #4162 ) ) ;
#2420=VERTEX_POINT ( 'NONE', #6046 ) ;
#2429=ORIENTED_EDGE ( 'NONE', *, *, #88, .T. ) ;
#2440=FACE_OUTER_BOUND ( 'NONE', #8159, .T. ) ;
#2444=EDGE_CURVE ( 'NONE', #2553, #7873, #188, .T. ) ;
#2445=VERTEX_POINT ( 'NONE', #4767 ) ;
#2456=EDGE_LOOP ( 'NONE', ( #1307, #2675 ) ) ;
#2461=VERTEX_POINT ( 'NONE', #2897 ) ;
#2464=DIRECTION ( 'NONE',  ( 0.000000000000000000, 0.000000000000000000, 1.000000000000000000 ) ) ;
#2473=CARTESIAN_POINT ( 'NONE',  ( -3.499085248937321868, -6.067035836480215494, 8.008459478482038207 ) ) ;
#2474=CARTESIAN_POINT ( 'NONE',  ( 1.810035846748221600, 6.765851833681423066, 8.002237581049140402 ) ) ;
#2503=CARTESIAN_POINT ( 'NONE',  ( 9.020562075079396891E-14, 10.00000000000000000, 729.2499999999977263 ) ) ;
#2505=LINE ( 'NONE', #627, #5061 ) ;
#2509=VECTOR ( 'NONE', #5743, 1000.000000000000000 ) ;
#2512=ORIENTED_EDGE ( 'NONE', *, *, #725, .T. ) ;
#2513=VERTEX_POINT ( 'NONE', #947 ) ;
#2514=CIRCLE ( 'NONE', #5043, 2.149999999999995470 ) ;
#2521=CARTESIAN_POINT ( 'NONE',  ( -1.813645741666879641, -6.764847328847696240, 8.002246981198915421 ) ) ;
#2534=DIRECTION ( 'NONE',  ( -0.000000000000000000, 1.000000000000000000, -0.000000000000000000 ) ) ;
#2553=VERTEX_POINT ( 'NONE', #988 ) ;
#2561=EDGE_CURVE ( 'NONE', #471, #2701, #2861, .T. ) ;
#2566=DIRECTION ( 'NONE',  ( 0.000000000000000000, 0.000000000000000000, -1.000000000000000000 ) ) ;
#2571=ORIENTED_EDGE ( 'NONE', *, *, #5994, .F. ) ;
#2572=CARTESIAN_POINT ( 'NONE',  ( -7.000000000000000000, 0.000000000000000000, 8.000000000000000000 ) ) ;
#2580=CARTESIAN_POINT ( 'NONE',  ( 0.000000000000000000, 0.000000000000000000, 0.000000000000000000 ) ) ;
#2584=CARTESIAN_POINT ( 'NONE',  ( 57.99999999999999289, 7.999999999999996447, 11.99999999999998934 ) ) ;
#2585=DIRECTION ( 'NONE',  ( -0.000000000000000000, -0.000000000000000000, 1.000000000000000000 ) ) ;
#2593=VERTEX_POINT ( 'NONE', #4858 ) ;
#2602=ORIENTED_EDGE ( 'NONE', *, *, #718, .F. ) ;
#2614=PLANE ( 'NONE',  #870 ) ;
#2617=LINE ( 'NONE', #1880, #4043 ) ;
#2624=CARTESIAN_POINT ( 'NONE',  ( 9.020562075079396891E-14, 10.00000000000000000, 8.000000000000007105 ) ) ;
#2629=CARTESIAN_POINT ( 'NONE',  ( -54.99999999999990052, -10.00000000000000000, 15.49999999999877254 ) ) ;
#2632=ORIENTED_EDGE ( 'NONE', *, *, #2211, .T. ) ;
#2633=MECHANICAL_DESIGN_GEOMETRIC_PRESENTATION_REPRESENTATION('',(#1557),#3295);
#2641=CARTESIAN_POINT ( 'NONE',  ( -5.271109574984434332, -4.628614387250548745, 8.019189290563998540 ) ) ;
#2642=AXIS2_PLACEMENT_3D ( 'NONE', #6817, #4792, #8055 ) ;
#2647=DIRECTION ( 'NONE',  ( 7.304098846218136639E-16, 0.000000000000000000, 1.000000000000000000 ) ) ;
#2664=CIRCLE ( 'NONE', #2642, 721.2499999999977263 ) ;
#2669=ORIENTED_EDGE ( 'NONE', *, *, #1889, .F. ) ;
#2674=ORIENTED_EDGE ( 'NONE', *, *, #776, .F. ) ;
#2675=ORIENTED_EDGE ( 'NONE', *, *, #253, .T. ) ;
#2682=ADVANCED_FACE ( 'NONE', ( #6312, #8170 ), #1152, .F. ) ;
#2688=CARTESIAN_POINT ( 'NONE',  ( 55.00000000000000000, 10.00000000000000000, 15.50000000000000355 ) ) ;
#2689=DIRECTION ( 'NONE',  ( 0.000000000000000000, 0.000000000000000000, 1.000000000000000000 ) ) ;
#2692=CARTESIAN_POINT ( 'NONE',  ( -60.00000000000000000, -10.00000000000000000, 20.00000000000000355 ) ) ;
#2699=ORIENTED_EDGE ( 'NONE', *, *, #485, .T. ) ;
#2701=VERTEX_POINT ( 'NONE', #6272 ) ;
#2709=EDGE_CURVE ( 'NONE', #5103, #4940, #1765, .T. ) ;
#2714=CARTESIAN_POINT ( 'NONE',  ( 5.566201872177863663, -4.269108285804360747, 8.021434216347806512 ) ) ;
#2724=CARTESIAN_POINT ( 'NONE',  ( 2.650000000000006573, 0.000000000000000000, 14.60000000000000142 ) ) ;
#2729=ORIENTED_EDGE ( 'NONE', *, *, #797, .T. ) ;
#2749=CARTESIAN_POINT ( 'NONE',  ( 2.253877478482040786, -6.643060962426256211, 8.003397232069101364 ) ) ;
#2768=CARTESIAN_POINT ( 'NONE',  ( 55.00000000000000000, 10.00000000000000000, 13.35000000000000853 ) ) ;
#2769=AXIS2_PLACEMENT_3D ( 'NONE', #4992, #7512, #2359 ) ;
#2775=EDGE_LOOP ( 'NONE', ( #7152, #1759, #4915, #2999, #1669 ) ) ;
#2784=DIRECTION ( 'NONE',  ( 0.000000000000000000, -1.000000000000000000, 0.000000000000000000 ) ) ;
#2787=LINE ( 'NONE', #5330, #5420 ) ;
#2788=CARTESIAN_POINT ( 'NONE',  ( -58.00000000000006395, 7.999999999999996447, 11.99999999999998934 ) ) ;
#2789=VECTOR ( 'NONE', #496, 1000.000000000000000 ) ;
#2794=VERTEX_POINT ( 'NONE', #7173 ) ;
#2797=CARTESIAN_POINT ( 'NONE',  ( 6.643161419842083859, -2.253695319827236254, 8.030573092606642760 ) ) ;
#2812=CARTESIAN_POINT ( 'NONE',  ( -52.00000000000006395, -8.000000000000003553, 11.99999999999998934 ) ) ;
#2816=AXIS2_PLACEMENT_3D ( 'NONE', #3749, #537, #8135 ) ;
#2833=ORIENTED_EDGE ( 'NONE', *, *, #7159, .F. ) ;
#2839=EDGE_CURVE ( 'NONE', #5534, #5475, #812, .T. ) ;
#2847=VERTEX_POINT ( 'NONE', #3992 ) ;
#2861=LINE ( 'NONE', #5329, #417 ) ;
#2863=CARTESIAN_POINT ( 'NONE',  ( -6.639644148827243519, 2.263345988190933689, 8.030540921233406237 ) ) ;
#2866=ORIENTED_EDGE ( 'NONE', *, *, #6995, .F. ) ;
#2870=DIRECTION ( 'NONE',  ( 0.000000000000000000, 0.000000000000000000, 1.000000000000000000 ) ) ;
#2871=CARTESIAN_POINT ( 'NONE',  ( 9.020562075079396891E-14, -10.00000000000000000, 8.000000000000007105 ) ) ;
#2877=ADVANCED_FACE ( 'NONE', ( #5206, #769, #5742 ), #3361, .F. ) ;
#2879=LINE ( 'NONE', #6565, #7033 ) ;
#2883=CIRCLE ( 'NONE', #8047, 2.149999999999995470 ) ;
#2897=CARTESIAN_POINT ( 'NONE',  ( -60.00000000000000000, -10.00000000000000000, 20.00000000000000355 ) ) ;
#2899=CARTESIAN_POINT ( 'NONE',  ( 60.00000000000014211, -10.00000000000000000, 10.50000000000006395 ) ) ;
#2900=VERTEX_POINT ( 'NONE', #2724 ) ;
#2901=AXIS2_PLACEMENT_3D ( 'NONE', #3178, #5052, #2464 ) ;
#2913=VECTOR ( 'NONE', #4311, 1000.000000000000000 ) ;
#2933=ORIENTED_EDGE ( 'NONE', *, *, #4581, .F. ) ;
#2935=CARTESIAN_POINT ( 'NONE',  ( 60.00000000000000711, -10.00000000000000000, 19.99999999999998224 ) ) ;
#2942=DIRECTION ( 'NONE',  ( -0.000000000000000000, -0.000000000000000000, 1.000000000000000000 ) ) ;
#2944=VERTEX_POINT ( 'NONE', #7954 ) ;
#2956=CARTESIAN_POINT ( 'NONE',  ( 55.00000000000000000, 10.00000000000000000, 13.35000000000000853 ) ) ;
#2958=ADVANCED_FACE ( 'NONE', ( #2271 ), #4681, .T. ) ;
#2960=VERTEX_POINT ( 'NONE', #2812 ) ;
#2976=FACE_OUTER_BOUND ( 'NONE', #579, .T. ) ;
#2992=DIRECTION ( 'NONE',  ( 0.000000000000000000, 1.000000000000000000, -0.000000000000000000 ) ) ;
#2999=ORIENTED_EDGE ( 'NONE', *, *, #6775, .F. ) ;
#3000=CARTESIAN_POINT ( 'NONE',  ( -54.99999999999990052, 10.00000000000000000, 15.49999999999877254 ) ) ;
#3005=CARTESIAN_POINT ( 'NONE',  ( 3.104279414096060119, 6.290759372240700031, 8.006556128919173787 ) ) ;
#3008=VERTEX_POINT ( 'NONE', #2184 ) ;
#3011=DIRECTION ( 'NONE',  ( 1.000000000000000000, 0.000000000000000000, 0.000000000000000000 ) ) ;
#3014=CIRCLE ( 'NONE', #755, 721.2499999999977263 ) ;
#3015=CARTESIAN_POINT ( 'NONE',  ( -3.469446951953613006E-15, 0.000000000000000000, 1.040834085586084257E-14 ) ) ;
#3031=CIRCLE ( 'NONE', #2769, 2.149999999999995470 ) ;
#3032=AXIS2_PLACEMENT_3D ( 'NONE', #5899, #125, #6553 ) ;
#3044=DIRECTION ( 'NONE',  ( 1.000000000000000000, 0.000000000000000000, 0.000000000000000000 ) ) ;
#3057=EDGE_CURVE ( 'NONE', #6951, #4508, #6625, .T. ) ;
#3065=CARTESIAN_POINT ( 'NONE',  ( -3.469446951953613006E-15, 0.000000000000000000, 20.00000000000000355 ) ) ;
#3070=DIRECTION ( 'NONE',  ( 0.000000000000000000, 0.000000000000000000, 1.000000000000000000 ) ) ;
#3093=VERTEX_POINT ( 'NONE', #1612 ) ;
#3095=FACE_OUTER_BOUND ( 'NONE', #2385, .T. ) ;
#3107=CARTESIAN_POINT ( 'NONE',  ( -58.00000000000006395, 7.999999999999996447, 19.99999999999998934 ) ) ;
#3128=EDGE_LOOP ( 'NONE', ( #5287, #2011, #2009, #3602 ) ) ;
#3135=ORIENTED_EDGE ( 'NONE', *, *, #6415, .T. ) ;
#3144=CYLINDRICAL_SURFACE ( 'NONE', #6769, 7.000000000000000000 ) ;
#3146=EDGE_CURVE ( 'NONE', #7631, #2513, #2883, .T. ) ;
#3149=VERTEX_POINT ( 'NONE', #1815 ) ;
#3156=FACE_BOUND ( 'NONE', #2417, .T. ) ;
#3169=LINE ( 'NONE', #2624, #4241 ) ;
#3170=PRODUCT_DEFINITION_CONTEXT ( 'detailed design', #927, 'design' ) ;
#3172=EDGE_LOOP ( 'NONE', ( #43, #6414, #5821, #8051 ) ) ;
#3173=ORIENTED_EDGE ( 'NONE', *, *, #7410, .T. ) ;
#3178=CARTESIAN_POINT ( 'NONE',  ( 55.00000000000000000, 10.00000000000000000, 15.50000000000000355 ) ) ;
#3200=ADVANCED_FACE ( 'NONE', ( #5109 ), #8191, .F. ) ;
#3229=EDGE_CURVE ( 'NONE', #2164, #4508, #7390, .T. ) ;
#3237=DIRECTION ( 'NONE',  ( 0.000000000000000000, 0.000000000000000000, 1.000000000000000000 ) ) ;
#3262=ORIENTED_EDGE ( 'NONE', *, *, #6255, .T. ) ;
#3270=( NAMED_UNIT ( * ) SI_UNIT ( $, .STERADIAN. ) SOLID_ANGLE_UNIT ( ) );
#3274=CYLINDRICAL_SURFACE ( 'NONE', #562, 2.650000000000002576 ) ;
#3285=CARTESIAN_POINT ( 'NONE',  ( -60.00000000000000000, 10.00000000000000000, 10.50000000000000000 ) ) ;
#3295=( GEOMETRIC_REPRESENTATION_CONTEXT ( 3 ) GLOBAL_UNCERTAINTY_ASSIGNED_CONTEXT ( ( #4292 ) ) GLOBAL_UNIT_ASSIGNED_CONTEXT ( ( #2347, #3822, #3270 ) ) REPRESENTATION_CONTEXT ( 'NONE', 'WORKASPACE' ) );
#3320=DIRECTION ( 'NONE',  ( 0.000000000000000000, 0.000000000000000000, 1.000000000000000000 ) ) ;
#3321=AXIS2_PLACEMENT_3D ( 'NONE', #8034, #3070, #6797 ) ;
#3326=AXIS2_PLACEMENT_3D ( 'NONE', #6531, #6077, #841 ) ;
#3342=ORIENTED_EDGE ( 'NONE', *, *, #2839, .T. ) ;
#3346=LINE ( 'NONE', #5873, #2351 ) ;
#3354=EDGE_CURVE ( 'NONE', #2847, #3149, #6586, .T. ) ;
#3361=PLANE ( 'NONE',  #7377 ) ;
#3367=EDGE_LOOP ( 'NONE', ( #3566, #7556, #1588, #2833 ) ) ;
#3368=LINE ( 'NONE', #193, #775 ) ;
#3371=ORIENTED_EDGE ( 'NONE', *, *, #3787, .T. ) ;
#3376=CARTESIAN_POINT ( 'NONE',  ( -52.00000000000006395, -8.000000000000001776, 20.00000000000000355 ) ) ;
#3377=CARTESIAN_POINT ( 'NONE',  ( 3.099070612933924274, -6.280812701381221608, 8.006629596177415209 ) ) ;
#3379=EDGE_CURVE ( 'NONE', #1461, #7794, #3346, .T. ) ;
#3386=CARTESIAN_POINT ( 'NONE',  ( -60.00000000000000000, 10.00000000000000000, 20.00000000000000355 ) ) ;
#3395=DIRECTION ( 'NONE',  ( 0.000000000000000000, 0.000000000000000000, -1.000000000000000000 ) ) ;
#3401=EDGE_LOOP ( 'NONE', ( #5943, #7911, #4628, #49, #1660 ) ) ;
#3404=CIRCLE ( 'NONE', #4601, 4.999999999999993783 ) ;
#3406=ADVANCED_FACE ( 'NONE', ( #2257 ), #458, .F. ) ;
#3408=PRODUCT_CONTEXT ( 'NONE', #4223, 'mechanical' ) ;
#3413=EDGE_CURVE ( 'NONE', #1727, #7382, #3014, .T. ) ;
#3417=AXIS2_PLACEMENT_3D ( 'NONE', #370, #6067, #6731 ) ;
#3453=DIRECTION ( 'NONE',  ( 0.000000000000000000, 1.000000000000000000, 0.000000000000000000 ) ) ;
#3473=EDGE_CURVE ( 'NONE', #6062, #2593, #2664, .T. ) ;
#3480=CARTESIAN_POINT ( 'NONE',  ( 60.00000000000000711, -10.00000000000000000, 19.99999999999998224 ) ) ;
#3500=CARTESIAN_POINT ( 'NONE',  ( 6.280460229959847318, -3.099761751707934998, 8.027336706075139716 ) ) ;
#3509=AXIS2_PLACEMENT_3D ( 'NONE', #2580, #5775, #7558 ) ;
#3512=ORIENTED_EDGE ( 'NONE', *, *, #398, .F. ) ;
#3513=ORIENTED_EDGE ( 'NONE', *, *, #6630, .F. ) ;
#3538=EDGE_CURVE ( 'NONE', #580, #7574, #1127, .T. ) ;
#3550=AXIS2_PLACEMENT_3D ( 'NONE', #3933, #751, #2133 ) ;
#3551=VECTOR ( 'NONE', #1562, 1000.000000000000000 ) ;
#3555=CIRCLE ( 'NONE', #1032, 2.149999999999995470 ) ;
#3556=CARTESIAN_POINT ( 'NONE',  ( 9.020562075079396891E-14, -10.00000000000000000, 729.2499999999977263 ) ) ;
#3563=EDGE_LOOP ( 'NONE', ( #6277, #7701 ) ) ;
#3566=ORIENTED_EDGE ( 'NONE', *, *, #253, .F. ) ;
#3569=VECTOR ( 'NONE', #5238, 1000.000000000000000 ) ;
#3579=AXIS2_PLACEMENT_3D ( 'NONE', #796, #865, #4665 ) ;
#3595=EDGE_CURVE ( 'NONE', #4814, #3913, #5628, .T. ) ;
#3596=AXIS2_PLACEMENT_3D ( 'NONE', #6967, #7601, #4561 ) ;
#3599=SHAPE_REPRESENTATION_RELATIONSHIP ( 'NONE' , 'NONE' ,  #1368, #4869 ) ;
#3602=ORIENTED_EDGE ( 'NONE', *, *, #292, .F. ) ;
#3606=CARTESIAN_POINT ( 'NONE',  ( -60.00000000000000000, 10.00000000000000000, 20.00000000000000355 ) ) ;
#3617=CARTESIAN_POINT ( 'NONE',  ( 4.999999999999990230, 0.000000000000000000, 20.00000000000000355 ) ) ;
#3622=EDGE_LOOP ( 'NONE', ( #5075, #6446, #3173, #625 ) ) ;
#3639=CARTESIAN_POINT ( 'NONE',  ( 5.948289146961254659, 3.697435614623359790, 8.024517386334258262 ) ) ;
#3642=AXIS2_PLACEMENT_3D ( 'NONE', #4189, #6765, #2357 ) ;
#3659=CARTESIAN_POINT ( 'NONE',  ( -4.264990453868429121, 5.569424739774936128, 8.012510174242292393 ) ) ;
#3666=EDGE_CURVE ( 'NONE', #6647, #7532, #1175, .T. ) ;
#3668=LINE ( 'NONE', #2956, #2789 ) ;
#3669=EDGE_CURVE ( 'NONE', #7873, #2445, #2366, .T. ) ;
#3672=CARTESIAN_POINT ( 'NONE',  ( -3.469446951953613006E-15, 0.000000000000000000, 20.00000000000000355 ) ) ;
#3678=FACE_BOUND ( 'NONE', #3172, .T. ) ;
#3680=ORIENTED_EDGE ( 'NONE', *, *, #3538, .T. ) ;
#3707=VECTOR ( 'NONE', #6102, 1000.000000000000000 ) ;
#3717=ORIENTED_EDGE ( 'NONE', *, *, #5660, .T. ) ;
#3721=CIRCLE ( 'NONE', #3857, 2.649999999999995026 ) ;
#3725=AXIS2_PLACEMENT_3D ( 'NONE', #1039, #2870, #5412 ) ;
#3735=PLANE ( 'NONE',  #2290 ) ;
#3741=CARTESIAN_POINT ( 'NONE',  ( 9.020562060468115204E-14, -7.000000000000000000, 7.999999999999977796 ) ) ;
#3742=CARTESIAN_POINT ( 'NONE',  ( -54.99999999999990052, 10.00000000000000000, 13.34999999999877573 ) ) ;
#3749=CARTESIAN_POINT ( 'NONE',  ( 52.00000000000000000, -8.000000000000003553, 11.99999999999998934 ) ) ;
#3754=ORIENTED_EDGE ( 'NONE', *, *, #718, .T. ) ;
#3760=CARTESIAN_POINT ( 'NONE',  ( -7.000000000000000000, 1.843750452292770530E-16, 8.033969604113661234 ) ) ;
#3761=CARTESIAN_POINT ( 'NONE',  ( 52.00000000000000000, -8.000000000000003553, 19.99999999999998934 ) ) ;
#3775=DIRECTION ( 'NONE',  ( -1.000000000000000000, 0.000000000000000000, 0.000000000000000000 ) ) ;
#3779=ORIENTED_EDGE ( 'NONE', *, *, #7159, .T. ) ;
#3786=DIRECTION ( 'NONE',  ( 0.000000000000000000, 0.000000000000000000, 1.000000000000000000 ) ) ;
#3787=EDGE_CURVE ( 'NONE', #2420, #5760, #3555, .T. ) ;
#3789=LINE ( 'NONE', #6972, #4580 ) ;
#3796=LINE ( 'NONE', #3285, #6231 ) ;
#3821=AXIS2_PLACEMENT_3D ( 'NONE', #8088, #8165, #3786 ) ;
#3822=( NAMED_UNIT ( * ) PLANE_ANGLE_UNIT ( ) SI_UNIT ( $, .RADIAN. ) );
#3826=DIRECTION ( 'NONE',  ( 0.000000000000000000, 0.000000000000000000, -1.000000000000000000 ) ) ;
#3836=EDGE_CURVE ( 'NONE', #8077, #4814, #4658, .T. ) ;
#3857=AXIS2_PLACEMENT_3D ( 'NONE', #3015, #7554, #4227 ) ;
#3875=EDGE_CURVE ( 'NONE', #5793, #7610, #2199, .T. ) ;
#3876=ORIENTED_EDGE ( 'NONE', *, *, #6630, .T. ) ;
#3883=DIRECTION ( 'NONE',  ( 0.000000000000000000, 0.000000000000000000, 1.000000000000000000 ) ) ;
#3887=AXIS2_PLACEMENT_3D ( 'NONE', #1832, #4359, #4907 ) ;
#3900=CARTESIAN_POINT ( 'NONE',  ( 52.00000000000000000, -8.000000000000003553, 11.99999999999998934 ) ) ;
#3902=CARTESIAN_POINT ( 'NONE',  ( 55.00000000000000000, 10.00000000000000000, 15.50000000000000355 ) ) ;
#3903=COLOUR_RGB ( '', 0.40784314, 0.44705882, 0.49803922) ;
#3913=VERTEX_POINT ( 'NONE', #361 ) ;
#3921=AXIS2_PLACEMENT_3D ( 'NONE', #1448, #262, #5853 ) ;
#3929=EDGE_LOOP ( 'NONE', ( #8122, #2729, #5371, #7502 ) ) ;
#3933=CARTESIAN_POINT ( 'NONE',  ( -54.99999999999990052, -10.00000000000000000, 15.49999999999877254 ) ) ;
#3942=CARTESIAN_POINT ( 'NONE',  ( 0.000000000000000000, 0.000000000000000000, 0.000000000000000000 ) ) ;
#3963=ORIENTED_EDGE ( 'NONE', *, *, #4149, .T. ) ;
#3965=VECTOR ( 'NONE', #2585, 1000.000000000000000 ) ;
#3977=AXIS2_PLACEMENT_3D ( 'NONE', #1771, #1091, #5636 ) ;
#3992=CARTESIAN_POINT ( 'NONE',  ( -54.99999999999990052, -10.00000000000000000, 17.64999999999876223 ) ) ;
#4002=EDGE_LOOP ( 'NONE', ( #4134, #7109, #3512, #864 ) ) ;
#4005=CARTESIAN_POINT ( 'NONE',  ( 7.000000000000000000, 8.572527594031473190E-16, 8.000000000000000000 ) ) ;
#4006=PLANE ( 'NONE',  #3032 ) ;
#4013=EDGE_CURVE ( 'NONE', #7532, #2900, #1209, .T. ) ;
#4021=DIRECTION ( 'NONE',  ( -0.000000000000000000, 1.000000000000000000, -0.000000000000000000 ) ) ;
#4025=ORIENTED_EDGE ( 'NONE', *, *, #2391, .F. ) ;
#4034=EDGE_CURVE ( 'NONE', #2847, #7631, #7132, .T. ) ;
#4037=LINE ( 'NONE', #4005, #4894 ) ;
#4043=VECTOR ( 'NONE', #6933, 1000.000000000000000 ) ;
#4054=CARTESIAN_POINT ( 'NONE',  ( 6.631756180578551430, 2.252199472339280195, 8.030486436084467883 ) ) ;
#4070=LINE ( 'NONE', #7914, #7277 ) ;
#4079=FACE_OUTER_BOUND ( 'NONE', #6981, .T. ) ;
#4089=( LENGTH_UNIT ( ) NAMED_UNIT ( * ) SI_UNIT ( .MILLI., .METRE. ) );
#4094=LINE ( 'NONE', #3386, #4954 ) ;
#4103=DIRECTION ( 'NONE',  ( -0.000000000000000000, -1.000000000000000000, -0.000000000000000000 ) ) ;
#4108=AXIS2_PLACEMENT_3D ( 'NONE', #3000, #8067, #2388 ) ;
#4116=CARTESIAN_POINT ( 'NONE',  ( -2.466926498672807888, 6.554919675146932079, 8.004187704512341739 ) ) ;
#4121=EDGE_LOOP ( 'NONE', ( #7178, #1896, #736, #6086 ) ) ;
#4134=ORIENTED_EDGE ( 'NONE', *, *, #50, .T. ) ;
#4138=CARTESIAN_POINT ( 'NONE',  ( 0.000000000000000000, 0.000000000000000000, 8.000000000000000000 ) ) ;
#4140=FACE_OUTER_BOUND ( 'NONE', #4803, .T. ) ;
#4147=EDGE_CURVE ( 'NONE', #2960, #5044, #7213, .T. ) ;
#4149=EDGE_CURVE ( 'NONE', #2794, #5782, #4387, .T. ) ;
#4155=CARTESIAN_POINT ( 'NONE',  ( -7.000000000000000000, 1.843750452292770530E-16, 8.033969604113661234 ) ) ;
#4162=ORIENTED_EDGE ( 'NONE', *, *, #3666, .T. ) ;
#4174=CARTESIAN_POINT ( 'NONE',  ( -6.075269275428587967, -3.507208453717142849, 8.025542426815230002 ) ) ;
#4182=PLANE ( 'NONE',  #4512 ) ;
#4189=CARTESIAN_POINT ( 'NONE',  ( 55.00000000000000000, -10.00000000000000000, 15.50000000000000355 ) ) ;
#4208=CYLINDRICAL_SURFACE ( 'NONE', #4108, 2.149999999999995470 ) ;
#4223=APPLICATION_CONTEXT ( 'automotive_design' ) ;
#4227=DIRECTION ( 'NONE',  ( 1.000000000000000000, 0.000000000000000000, 0.000000000000000000 ) ) ;
#4231=ORIENTED_EDGE ( 'NONE', *, *, #111, .T. ) ;
#4233=CIRCLE ( 'NONE', #7687, 2.650000000000010125 ) ;
#4239=CARTESIAN_POINT ( 'NONE',  ( -0.4613443011311406106, 7.000000000000005329, 8.000000000000021316 ) ) ;
#4241=VECTOR ( 'NONE', #5749, 1000.000000000000000 ) ;
#4245=ORIENTED_EDGE ( 'NONE', *, *, #2036, .F. ) ;
#4255=VECTOR ( 'NONE', #1361, 1000.000000000000000 ) ;
#4260=CARTESIAN_POINT ( 'NONE',  ( -58.00000000000006395, -8.000000000000003553, 11.99999999999998934 ) ) ;
#4266=VERTEX_POINT ( 'NONE', #8127 ) ;
#4274=ADVANCED_FACE ( 'NONE', ( #2440 ), #4985, .F. ) ;
#4275=ORIENTED_EDGE ( 'NONE', *, *, #3229, .T. ) ;
#4276=ADVANCED_FACE ( 'NONE', ( #4441, #1915 ), #8033, .F. ) ;
#4278=DIRECTION ( 'NONE',  ( -0.000000000000000000, -0.000000000000000000, 1.000000000000000000 ) ) ;
#4282=CARTESIAN_POINT ( 'NONE',  ( 9.020562070449730010E-14, 7.000000000000000000, 8.000000000000058620 ) ) ;
#4292=UNCERTAINTY_MEASURE_WITH_UNIT (LENGTH_MEASURE( 1.000000000000000082E-05 ), #2347, 'distance_accuracy_value', 'NONE');
#4297=CARTESIAN_POINT ( 'NONE',  ( -4.999999999999997335, 6.123233995736758394E-16, 20.00000000000000355 ) ) ;
#4300=CARTESIAN_POINT ( 'NONE',  ( -6.765702216007799308, -1.810551654344674688, 8.031730529104347482 ) ) ;
#4305=ORIENTED_EDGE ( 'NONE', *, *, #3473, .F. ) ;
#4310=DIRECTION ( 'NONE',  ( 0.000000000000000000, 0.000000000000000000, 1.000000000000000000 ) ) ;
#4311=DIRECTION ( 'NONE',  ( -0.000000000000000000, 1.000000000000000000, -0.000000000000000000 ) ) ;
#4317=FACE_OUTER_BOUND ( 'NONE', #8052, .T. ) ;
#4331=ORIENTED_EDGE ( 'NONE', *, *, #7410, .F. ) ;
#4332=FACE_OUTER_BOUND ( 'NONE', #3622, .T. ) ;
#4336=ORIENTED_EDGE ( 'NONE', *, *, #7686, .T. ) ;
#4337=FACE_BOUND ( 'NONE', #5503, .T. ) ;
#4343=CARTESIAN_POINT ( 'NONE',  ( 6.477744019519650287, 2.682274772516526351, 8.029074116683069917 ) ) ;
#4359=DIRECTION ( 'NONE',  ( -0.000000000000000000, -0.000000000000000000, 1.000000000000000000 ) ) ;
#4369=VERTEX_POINT ( 'NONE', #3741 ) ;
#4372=VECTOR ( 'NONE', #4278, 1000.000000000000000 ) ;
#4387=CIRCLE ( 'NONE', #249, 2.149999999999999023 ) ;
#4390=CARTESIAN_POINT ( 'NONE',  ( 55.00000000000000000, -8.000000000000001776, 15.50000000000000355 ) ) ;
#4394=AXIS2_PLACEMENT_3D ( 'NONE', #831, #5257, #5945 ) ;
#4395=CARTESIAN_POINT ( 'NONE',  ( 6.067105206393708094, 3.498950914359637121, 8.025510423632917778 ) ) ;
#4403=FACE_OUTER_BOUND ( 'NONE', #4418, .T. ) ;
#4406=DIRECTION ( 'NONE',  ( 0.000000000000000000, 1.000000000000000000, 0.000000000000000000 ) ) ;
#4418=EDGE_LOOP ( 'NONE', ( #2933, #7523, #2190, #4464 ) ) ;
#4421=LINE ( 'NONE', #6947, #1342 ) ;
#4427=ORIENTED_EDGE ( 'NONE', *, *, #6931, .F. ) ;
#4439=CARTESIAN_POINT ( 'NONE',  ( -58.00000000000006395, -8.000000000000003553, 11.99999999999998934 ) ) ;
#4441=FACE_BOUND ( 'NONE', #7416, .T. ) ;
#4444=DIRECTION ( 'NONE',  ( 0.000000000000000000, 0.000000000000000000, 1.000000000000000000 ) ) ;
#4452=ADVANCED_FACE ( 'NONE', ( #4317 ), #4991, .F. ) ;
#4458=LINE ( 'NONE', #6906, #1988 ) ;
#4463=ORIENTED_EDGE ( 'NONE', *, *, #2391, .T. ) ;
#4464=ORIENTED_EDGE ( 'NONE', *, *, #2444, .F. ) ;
#4471=CARTESIAN_POINT ( 'NONE',  ( -1.588954872702794896, -6.821165568473427143, 8.001714880650744988 ) ) ;
#4490=CIRCLE ( 'NONE', #1839, 721.2499999999977263 ) ;
#4498=DIRECTION ( 'NONE',  ( 1.000000000000000000, 0.000000000000000000, 0.000000000000000000 ) ) ;
#4499=DIRECTION ( 'NONE',  ( -0.000000000000000000, 1.000000000000000000, -0.000000000000000000 ) ) ;
#4504=VECTOR ( 'NONE', #5282, 1000.000000000000000 ) ;
#4508=VERTEX_POINT ( 'NONE', #1205 ) ;
#4510=AXIS2_PLACEMENT_3D ( 'NONE', #4565, #7094, #7172 ) ;
#4512=AXIS2_PLACEMENT_3D ( 'NONE', #3606, #6579, #6134 ) ;
#4516=CARTESIAN_POINT ( 'NONE',  ( 0.000000000000000000, 0.000000000000000000, 8.000000000000000000 ) ) ;
#4522=DIRECTION ( 'NONE',  ( 0.000000000000000000, -1.000000000000000000, 0.000000000000000000 ) ) ;
#4549=VECTOR ( 'NONE', #7959, 1000.000000000000000 ) ;
#4552=DIRECTION ( 'NONE',  ( -0.000000000000000000, 1.000000000000000000, -0.000000000000000000 ) ) ;
#4557=FACE_OUTER_BOUND ( 'NONE', #3401, .T. ) ;
#4560=LINE ( 'NONE', #805, #120 ) ;
#4561=DIRECTION ( 'NONE',  ( 1.000000000000000000, 0.000000000000000000, -0.000000000000000000 ) ) ;
#4565=CARTESIAN_POINT ( 'NONE',  ( -52.00000000000006395, -8.000000000000003553, 11.99999999999998934 ) ) ;
#4580=VECTOR ( 'NONE', #4406, 1000.000000000000000 ) ;
#4581=EDGE_CURVE ( 'NONE', #3093, #2553, #2514, .T. ) ;
#4595=AXIS2_PLACEMENT_3D ( 'NONE', #3672, #503, #3044 ) ;
#4601=AXIS2_PLACEMENT_3D ( 'NONE', #399, #2942, #2316 ) ;
#4604=CARTESIAN_POINT ( 'NONE',  ( 57.99999999999999289, -8.000000000000003553, 11.99999999999998934 ) ) ;
#4606=FACE_OUTER_BOUND ( 'NONE', #1101, .T. ) ;
#4612=EDGE_LOOP ( 'NONE', ( #5447, #7305, #8092, #747 ) ) ;
#4616=SHAPE_DEFINITION_REPRESENTATION ( #7426, #1368 ) ;
#4622=PLANE ( 'NONE',  #3579 ) ;
#4623=CARTESIAN_POINT ( 'NONE',  ( 7.000000000000000000, 8.572527785734883977E-16, 8.033969604113771368 ) ) ;
#4628=ORIENTED_EDGE ( 'NONE', *, *, #1282, .F. ) ;
#4640=DIRECTION ( 'NONE',  ( -0.000000000000000000, 1.000000000000000000, -0.000000000000000000 ) ) ;
#4646=CARTESIAN_POINT ( 'NONE',  ( -54.99999999999990052, 10.00000000000000000, 17.64999999999876579 ) ) ;
#4647=CARTESIAN_POINT ( 'NONE',  ( 55.00000000000000000, 10.00000000000000000, 17.64999999999999858 ) ) ;
#4652=EDGE_LOOP ( 'NONE', ( #4275, #2068 ) ) ;
#4658=LINE ( 'NONE', #2788, #7137 ) ;
#4665=DIRECTION ( 'NONE',  ( 0.000000000000000000, -0.000000000000000000, -1.000000000000000000 ) ) ;
#4666=CARTESIAN_POINT ( 'NONE',  ( 3.504480373706772234, -6.063947902487814012, 8.008485521361658144 ) ) ;
#4677=CARTESIAN_POINT ( 'NONE',  ( 6.821338123897841221, 1.588166687390477616, 8.032256283446461254 ) ) ;
#4678=ORIENTED_EDGE ( 'NONE', *, *, #6865, .T. ) ;
#4679=CARTESIAN_POINT ( 'NONE',  ( -52.00000000000006395, 7.999999999999996447, 11.99999999999998934 ) ) ;
#4681=CYLINDRICAL_SURFACE ( 'NONE', #1421, 7.000000000000000000 ) ;
#4683=CARTESIAN_POINT ( 'NONE',  ( 52.00000000000000000, -8.000000000000003553, 19.99999999999998934 ) ) ;
#4685=DIRECTION ( 'NONE',  ( 0.000000000000000000, 0.000000000000000000, 1.000000000000000000 ) ) ;
#4704=CARTESIAN_POINT ( 'NONE',  ( 6.379742460914609836, -2.889908336535204292, 8.028210883294187639 ) ) ;
#4717=DIRECTION ( 'NONE',  ( 0.000000000000000000, 1.000000000000000000, -0.000000000000000000 ) ) ;
#4718=DIRECTION ( 'NONE',  ( -0.000000000000000000, -0.000000000000000000, -1.000000000000000000 ) ) ;
#4722=DIRECTION ( 'NONE',  ( 0.000000000000000000, 1.000000000000000000, -0.000000000000000000 ) ) ;
#4734=ORIENTED_EDGE ( 'NONE', *, *, #4034, .T. ) ;
#4745=VECTOR ( 'NONE', #1690, 1000.000000000000000 ) ;
#4754=AXIS2_PLACEMENT_3D ( 'NONE', #142, #95, #2647 ) ;
#4755=AXIS2_PLACEMENT_3D ( 'NONE', #4984, #7505, #1993 ) ;
#4756=EDGE_CURVE ( 'NONE', #5567, #2900, #4233, .T. ) ;
#4764=CARTESIAN_POINT ( 'NONE',  ( 60.00000000000014211, 10.00000000000000000, 10.50000000000006395 ) ) ;
#4767=CARTESIAN_POINT ( 'NONE',  ( 55.00000000000000000, 10.00000000000000000, 13.35000000000000497 ) ) ;
#4769=CIRCLE ( 'NONE', #6614, 2.149999999999999023 ) ;
#4775=AXIS2_PLACEMENT_3D ( 'NONE', #6965, #1780, #4310 ) ;
#4785=EDGE_CURVE ( 'NONE', #5103, #6416, #6825, .T. ) ;
#4789=ADVANCED_FACE ( 'NONE', ( #7406, #4337, #4879 ), #7496, .T. ) ;
#4791=CARTESIAN_POINT ( 'NONE',  ( 6.954242511297643148, -0.9206211859927554420, 8.033521398158129045 ) ) ;
#4792=DIRECTION ( 'NONE',  ( 0.000000000000000000, 1.000000000000000000, -0.000000000000000000 ) ) ;
#4794=EDGE_LOOP ( 'NONE', ( #8176, #4305, #943, #5869, #1381, #2395, #2632 ) ) ;
#4796=B_SPLINE_CURVE_WITH_KNOTS ( 'NONE', 3,
 ( #4282, #4239, #5493, #6807, #1116, #5575, #4116, #8004, #6768, #3659, #7261, #2287, #1581, #6016, #6682, #4821, #7349, #2863, #7918, #7311, #1625, #4155 ),
 .UNSPECIFIED., .F., .F.,
 ( 4, 2, 2, 2, 2, 2, 2, 2, 2, 2, 4 ),
 ( 0.03283134218946166805, 0.03419813915831548812, 0.03488153764274239815, 0.03556493612716930819, 0.03693173309602312826, 0.03829853006487694833, 0.03966532703373076840, 0.04034872551815767844, 0.04103212400258458847, 0.04239892097143841548, 0.04376571794029223555 ),
 .UNSPECIFIED. ) ;
#4803=EDGE_LOOP ( 'NONE', ( #2235, #1331, #3717, #5204, #2512, #7427, #2602 ) ) ;
#4808=FACE_OUTER_BOUND ( 'NONE', #1430, .T. ) ;
#4814=VERTEX_POINT ( 'NONE', #4260 ) ;
#4818=ADVANCED_FACE ( 'NONE', ( #6076 ), #6786, .F. ) ;
#4820=B_SPLINE_CURVE_WITH_KNOTS ( 'NONE', 3,
 ( #2265, #426, #8070, #382, #4300, #6828, #7327, #1645, #4174, #8154, #2641, #2028, #5190, #7709, #2473, #1399, #5070, #7044, #2521, #4471, #1986, #1313, #8194 ),
 .UNSPECIFIED., .F., .F.,
 ( 4, 2, 2, 2, 2, 2, 2, 2, 1, 2, 2, 4 ),
 ( 6.815276097578277091E-20, 0.001368142784595155264, 0.002052214176892732354, 0.002736285569190309661, 0.004104428353785464709, 0.005472571138380617588, 0.006840713922975770467, 0.007524785315273349075, 0.008208856707570925948, 0.008892928099868503689, 0.009576999492166081429, 0.01094514227676123691 ),
 .UNSPECIFIED. ) ;
#4821=CARTESIAN_POINT ( 'NONE',  ( -6.279904204137568335, 3.100863108398094425, 8.027331884377945315 ) ) ;
#4834=EDGE_LOOP ( 'NONE', ( #7316, #1275, #746, #3963 ) ) ;
#4841=FACE_BOUND ( 'NONE', #315, .T. ) ;
#4850=ADVANCED_FACE ( 'NONE', ( #3095 ), #4208, .F. ) ;
#4853=CARTESIAN_POINT ( 'NONE',  ( -54.99999999999990052, 10.00000000000000000, 15.49999999999877254 ) ) ;
#4857=CYLINDRICAL_SURFACE ( 'NONE', #7412, 2.149999999999995470 ) ;
#4858=CARTESIAN_POINT ( 'NONE',  ( 9.020562075079396891E-14, 10.00000000000000000, 8.000000000000007105 ) ) ;
#4869=ADVANCED_BREP_SHAPE_REPRESENTATION ( '', ( #6918, #1587 ), #2170 ) ;
#4879=FACE_OUTER_BOUND ( 'NONE', #2775, .T. ) ;
#4885=CARTESIAN_POINT ( 'NONE',  ( 2.250597875665110603, 6.632329153766082008, 8.003477766920562786 ) ) ;
#4890=SURFACE_STYLE_USAGE ( .BOTH. , #2398 ) ;
#4894=VECTOR ( 'NONE', #6587, 1000.000000000000000 ) ;
#4900=VERTEX_POINT ( 'NONE', #5107 ) ;
#4907=DIRECTION ( 'NONE',  ( 1.000000000000000000, 0.000000000000000000, 0.000000000000000000 ) ) ;
#4914=VECTOR ( 'NONE', #4685, 1000.000000000000000 ) ;
#4915=ORIENTED_EDGE ( 'NONE', *, *, #485, .F. ) ;
#4920=CARTESIAN_POINT ( 'NONE',  ( -52.00000000000006395, 7.999999999999996447, 19.99999999999998934 ) ) ;
#4929=ORIENTED_EDGE ( 'NONE', *, *, #3669, .F. ) ;
#4937=EDGE_CURVE ( 'NONE', #2420, #5782, #6291, .T. ) ;
#4940=VERTEX_POINT ( 'NONE', #5011 ) ;
#4942=DIRECTION ( 'NONE',  ( 1.000000000000000000, 0.000000000000000000, 0.000000000000000000 ) ) ;
#4946=DIRECTION ( 'NONE',  ( 0.000000000000000000, 0.000000000000000000, 1.000000000000000000 ) ) ;
#4954=VECTOR ( 'NONE', #929, 1000.000000000000000 ) ;
#4984=CARTESIAN_POINT ( 'NONE',  ( -3.469446951953613006E-15, 0.000000000000000000, 14.60000000000000142 ) ) ;
#4985=PLANE ( 'NONE',  #130 ) ;
#4986=PLANE ( 'NONE',  #3321 ) ;
#4991=PLANE ( 'NONE',  #4754 ) ;
#4992=CARTESIAN_POINT ( 'NONE',  ( 55.00000000000000000, 7.999999999999996447, 15.50000000000000355 ) ) ;
#5002=CYLINDRICAL_SURFACE ( 'NONE', #7799, 721.2499999999977263 ) ;
#5008=AXIS2_PLACEMENT_3D ( 'NONE', #5851, #1445, #4444 ) ;
#5011=CARTESIAN_POINT ( 'NONE',  ( 4.999999999999990230, 0.000000000000000000, 14.60000000000000142 ) ) ;
#5016=DIRECTION ( 'NONE',  ( 0.000000000000000000, 0.000000000000000000, -1.000000000000000000 ) ) ;
#5043=AXIS2_PLACEMENT_3D ( 'NONE', #923, #7858, #873 ) ;
#5044=VERTEX_POINT ( 'NONE', #3376 ) ;
#5052=DIRECTION ( 'NONE',  ( -0.000000000000000000, 1.000000000000000000, -0.000000000000000000 ) ) ;
#5061=VECTOR ( 'NONE', #2148, 1000.000000000000000 ) ;
#5070=CARTESIAN_POINT ( 'NONE',  ( -2.681845249323461911, -6.477919090352733278, 8.004893738113867840 ) ) ;
#5074=ORIENTED_EDGE ( 'NONE', *, *, #7008, .F. ) ;
#5075=ORIENTED_EDGE ( 'NONE', *, *, #2709, .F. ) ;
#5077=FILL_AREA_STYLE_COLOUR ( '', #5283 ) ;
#5085=CARTESIAN_POINT ( 'NONE',  ( -54.99999999999990052, 10.00000000000000000, 17.64999999999876579 ) ) ;
#5095=AXIS2_PLACEMENT_3D ( 'NONE', #816, #4722, #3395 ) ;
#5103=VERTEX_POINT ( 'NONE', #5871 ) ;
#5107=CARTESIAN_POINT ( 'NONE',  ( 9.020562070449730010E-14, 7.000000000000000000, 8.000000000000058620 ) ) ;
#5109=FACE_OUTER_BOUND ( 'NONE', #1068, .T. ) ;
#5115=CARTESIAN_POINT ( 'NONE',  ( -54.99999999999990052, 10.00000000000000000, 15.49999999999877254 ) ) ;
#5132=ORIENTED_EDGE ( 'NONE', *, *, #3379, .T. ) ;
#5133=ORIENTED_EDGE ( 'NONE', *, *, #838, .T. ) ;
#5139=ADVANCED_FACE ( 'NONE', ( #1544, #4079 ), #4622, .F. ) ;
#5144=CARTESIAN_POINT ( 'NONE',  ( -54.99999999999990052, 10.00000000000000000, 13.34999999999877573 ) ) ;
#5146=DIRECTION ( 'NONE',  ( 0.000000000000000000, 0.000000000000000000, -1.000000000000000000 ) ) ;
#5152=DIRECTION ( 'NONE',  ( 0.000000000000000000, 0.000000000000000000, 1.000000000000000000 ) ) ;
#5172=CARTESIAN_POINT ( 'NONE',  ( 7.000000000000000000, 8.572527785734883977E-16, 8.033969604113771368 ) ) ;
#5190=CARTESIAN_POINT ( 'NONE',  ( -4.272249441377914181, -5.564160999819695697, 8.012551623441856563 ) ) ;
#5204=ORIENTED_EDGE ( 'NONE', *, *, #1282, .T. ) ;
#5206=FACE_BOUND ( 'NONE', #6072, .T. ) ;
#5208=DIRECTION ( 'NONE',  ( 1.000000000000000000, 0.000000000000000000, 0.000000000000000000 ) ) ;
#5233=STYLED_ITEM ( 'NONE', ( #5956 ), #4869 ) ;
#5235=EDGE_CURVE ( 'NONE', #3008, #4266, #5833, .T. ) ;
#5238=DIRECTION ( 'NONE',  ( 0.000000000000000000, 1.000000000000000000, 0.000000000000000000 ) ) ;
#5239=DIRECTION ( 'NONE',  ( 0.000000000000000000, -1.000000000000000000, 0.000000000000000000 ) ) ;
#5247=VERTEX_POINT ( 'NONE', #1083 ) ;
#5257=DIRECTION ( 'NONE',  ( -0.000000000000000000, -0.000000000000000000, 1.000000000000000000 ) ) ;
#5277=ORIENTED_EDGE ( 'NONE', *, *, #6204, .F. ) ;
#5282=DIRECTION ( 'NONE',  ( 0.000000000000000000, 1.000000000000000000, 0.000000000000000000 ) ) ;
#5283=COLOUR_RGB ( '', 0.40784314, 0.44705882, 0.49803922) ;
#5284=CARTESIAN_POINT ( 'NONE',  ( 52.00000000000000000, 7.999999999999996447, 11.99999999999998934 ) ) ;
#5285=DIRECTION ( 'NONE',  ( 0.000000000000000000, 0.000000000000000000, 1.000000000000000000 ) ) ;
#5287=ORIENTED_EDGE ( 'NONE', *, *, #3787, .F. ) ;
#5288=EDGE_LOOP ( 'NONE', ( #1393, #1942 ) ) ;
#5292=CARTESIAN_POINT ( 'NONE',  ( 2.889328000935821095, -6.379995247853900153, 8.005756244325109350 ) ) ;
#5315=DIRECTION ( 'NONE',  ( -0.000000000000000000, 1.000000000000000000, -0.000000000000000000 ) ) ;
#5316=DIRECTION ( 'NONE',  ( 0.000000000000000000, 0.000000000000000000, -1.000000000000000000 ) ) ;
#5329=CARTESIAN_POINT ( 'NONE',  ( 57.99999999999999289, -8.000000000000003553, 11.99999999999998934 ) ) ;
#5330=CARTESIAN_POINT ( 'NONE',  ( -60.00000000000000000, 10.00000000000000000, 20.00000000000000355 ) ) ;
#5351=EDGE_CURVE ( 'NONE', #5475, #471, #4458, .T. ) ;
#5362=EDGE_LOOP ( 'NONE', ( #1020, #7693 ) ) ;
#5370=VERTEX_POINT ( 'NONE', #5172 ) ;
#5371=ORIENTED_EDGE ( 'NONE', *, *, #3146, .F. ) ;
#5375=ADVANCED_FACE ( 'NONE', ( #585 ), #5002, .T. ) ;
#5386=VERTEX_POINT ( 'NONE', #3760 ) ;
#5403=LINE ( 'NONE', #7345, #4372 ) ;
#5412=DIRECTION ( 'NONE',  ( 1.000000000000000000, 0.000000000000000000, 0.000000000000000000 ) ) ;
#5415=AXIS2_PLACEMENT_3D ( 'NONE', #4390, #1982, #2566 ) ;
#5420=VECTOR ( 'NONE', #7844, 1000.000000000000000 ) ;
#5426=CARTESIAN_POINT ( 'NONE',  ( 7.000000000000000000, 8.572527785734883977E-16, 8.033969604113771368 ) ) ;
#5427=VECTOR ( 'NONE', #6123, 1000.000000000000000 ) ;
#5434=VECTOR ( 'NONE', #4552, 1000.000000000000000 ) ;
#5447=ORIENTED_EDGE ( 'NONE', *, *, #50, .F. ) ;
#5449=LINE ( 'NONE', #481, #3707 ) ;
#5472=( NAMED_UNIT ( * ) PLANE_ANGLE_UNIT ( ) SI_UNIT ( $, .RADIAN. ) );
#5475=VERTEX_POINT ( 'NONE', #1423 ) ;
#5493=CARTESIAN_POINT ( 'NONE',  ( -0.9176763012970977629, 6.954530811262681134, 8.000445331782056968 ) ) ;
#5494=EDGE_LOOP ( 'NONE', ( #999, #4245, #4025, #6511 ) ) ;
#5503=EDGE_LOOP ( 'NONE', ( #162, #6113 ) ) ;
#5509=DIRECTION ( 'NONE',  ( 1.000000000000000000, 0.000000000000000000, 0.000000000000000000 ) ) ;
#5526=ADVANCED_FACE ( 'NONE', ( #7143 ), #4006, .T. ) ;
#5534=VERTEX_POINT ( 'NONE', #5284 ) ;
#5549=VECTOR ( 'NONE', #5645, 1000.000000000000000 ) ;
#5553=EDGE_CURVE ( 'NONE', #6876, #7471, #2787, .T. ) ;
#5567=VERTEX_POINT ( 'NONE', #2050 ) ;
#5575=CARTESIAN_POINT ( 'NONE',  ( -2.248460506220263166, 6.633023922978178888, 8.003471350439957277 ) ) ;
#5577=CIRCLE ( 'NONE', #8078, 2.149999999999995470 ) ;
#5595=DIRECTION ( 'NONE',  ( 0.000000000000000000, -0.000000000000000000, -1.000000000000000000 ) ) ;
#5628=LINE ( 'NONE', #497, #6078 ) ;
#5636=DIRECTION ( 'NONE',  ( 0.000000000000000000, 0.000000000000000000, 1.000000000000000000 ) ) ;
#5644=CIRCLE ( 'NONE', #3642, 2.149999999999992362 ) ;
#5645=DIRECTION ( 'NONE',  ( 0.000000000000000000, -1.000000000000000000, 0.000000000000000000 ) ) ;
#5648=DIRECTION ( 'NONE',  ( -1.000000000000000000, 0.000000000000000000, 0.000000000000000000 ) ) ;
#5660=EDGE_CURVE ( 'NONE', #4900, #5386, #4796, .T. ) ;
#5669=DIRECTION ( 'NONE',  ( 0.000000000000000000, 0.000000000000000000, 1.000000000000000000 ) ) ;
#5680=DIRECTION ( 'NONE',  ( -0.000000000000000000, -0.000000000000000000, -1.000000000000000000 ) ) ;
#5682=ORIENTED_EDGE ( 'NONE', *, *, #6326, .F. ) ;
#5729=LINE ( 'NONE', #7083, #4255 ) ;
#5732=CARTESIAN_POINT ( 'NONE',  ( 55.00000000000000000, -10.00000000000000000, 13.35000000000001030 ) ) ;
#5736=DIRECTION ( 'NONE',  ( -0.000000000000000000, 1.000000000000000000, -0.000000000000000000 ) ) ;
#5737=DIRECTION ( 'NONE',  ( 0.000000000000000000, 1.000000000000000000, -0.000000000000000000 ) ) ;
#5742=FACE_OUTER_BOUND ( 'NONE', #545, .T. ) ;
#5743=DIRECTION ( 'NONE',  ( -0.000000000000000000, -1.000000000000000000, -0.000000000000000000 ) ) ;
#5748=PRODUCT_DEFINITION ( 'UNKNOWN', '', #289, #3170 ) ;
#5749=DIRECTION ( 'NONE',  ( -0.000000000000000000, -1.000000000000000000, -0.000000000000000000 ) ) ;
#5759=EDGE_CURVE ( 'NONE', #7471, #2461, #615, .T. ) ;
#5760=VERTEX_POINT ( 'NONE', #36 ) ;
#5772=CYLINDRICAL_SURFACE ( 'NONE', #5008, 2.149999999999995470 ) ;
#5775=DIRECTION ( 'NONE',  ( 0.000000000000000000, 0.000000000000000000, 1.000000000000000000 ) ) ;
#5782=VERTEX_POINT ( 'NONE', #664 ) ;
#5792=ORIENTED_EDGE ( 'NONE', *, *, #7733, .T. ) ;
#5793=VERTEX_POINT ( 'NONE', #2584 ) ;
#5807=CARTESIAN_POINT ( 'NONE',  ( -3.469446951953613006E-15, 0.000000000000000000, 20.00000000000000355 ) ) ;
#5821=ORIENTED_EDGE ( 'NONE', *, *, #88, .F. ) ;
#5826=AXIS2_PLACEMENT_3D ( 'NONE', #628, #6244, #8183 ) ;
#5832=ORIENTED_EDGE ( 'NONE', *, *, #3836, .F. ) ;
#5833=CIRCLE ( 'NONE', #3725, 7.000000000000000000 ) ;
#5848=LINE ( 'NONE', #3900, #1197 ) ;
#5851=CARTESIAN_POINT ( 'NONE',  ( 55.00000000000000000, 10.00000000000000000, 15.50000000000000355 ) ) ;
#5853=DIRECTION ( 'NONE',  ( -1.000000000000000000, 0.000000000000000000, -0.000000000000000000 ) ) ;
#5869=ORIENTED_EDGE ( 'NONE', *, *, #3413, .T. ) ;
#5871=CARTESIAN_POINT ( 'NONE',  ( -4.999999999999997335, 6.123233995736758394E-16, 14.60000000000000142 ) ) ;
#5873=CARTESIAN_POINT ( 'NONE',  ( 60.00000000000000711, 10.00000000000000000, 19.99999999999998224 ) ) ;
#5876=EDGE_CURVE ( 'NONE', #7622, #2701, #813, .T. ) ;
#5884=CYLINDRICAL_SURFACE ( 'NONE', #1628, 2.149999999999995470 ) ;
#5886=FACE_BOUND ( 'NONE', #1657, .T. ) ;
#5888=DIRECTION ( 'NONE',  ( 0.000000000000000000, -1.000000000000000000, 0.000000000000000000 ) ) ;
#5899=CARTESIAN_POINT ( 'NONE',  ( -110.0000000000000711, -3.212021572632693692E-15, 11.99999999999998934 ) ) ;
#5902=ADVANCED_FACE ( 'NONE', ( #4606 ), #7131, .F. ) ;
#5943=ORIENTED_EDGE ( 'NONE', *, *, #33, .F. ) ;
#5945=DIRECTION ( 'NONE',  ( 1.000000000000000000, 0.000000000000000000, 0.000000000000000000 ) ) ;
#5956=PRESENTATION_STYLE_ASSIGNMENT (( #335 ) ) ;
#5959=CARTESIAN_POINT ( 'NONE',  ( 55.00000000000000000, -10.00000000000000000, 17.64999999999999503 ) ) ;
#5961=PLANE ( 'NONE',  #3921 ) ;
#5986=CARTESIAN_POINT ( 'NONE',  ( 5.946271935299904499, -3.700516488397892712, 8.024501004382219804 ) ) ;
#5994=EDGE_CURVE ( 'NONE', #6062, #1727, #1613, .T. ) ;
#5997=FACE_BOUND ( 'NONE', #5288, .T. ) ;
#6004=CYLINDRICAL_SURFACE ( 'NONE', #7807, 721.2499999999977263 ) ;
#6013=LINE ( 'NONE', #7221, #4504 ) ;
#6016=CARTESIAN_POINT ( 'NONE',  ( -5.944181862675879557, 3.703975565927438041, 8.024483585023222787 ) ) ;
#6025=CARTESIAN_POINT ( 'NONE',  ( 0.4564736065166624668, -6.999999999999996447, 8.000000000000044409 ) ) ;
#6026=DIRECTION ( 'NONE',  ( 0.000000000000000000, 0.000000000000000000, 1.000000000000000000 ) ) ;
#6038=ORIENTED_EDGE ( 'NONE', *, *, #1318, .F. ) ;
#6046=CARTESIAN_POINT ( 'NONE',  ( -54.99999999999990052, 7.999999999999996447, 13.34999999999877573 ) ) ;
#6055=DIRECTION ( 'NONE',  ( -0.000000000000000000, 1.000000000000000000, -0.000000000000000000 ) ) ;
#6062=VERTEX_POINT ( 'NONE', #4764 ) ;
#6067=DIRECTION ( 'NONE',  ( -0.000000000000000000, -0.000000000000000000, 1.000000000000000000 ) ) ;
#6069=AXIS2_PLACEMENT_3D ( 'NONE', #8080, #4522, #7085 ) ;
#6072=EDGE_LOOP ( 'NONE', ( #4929, #1012 ) ) ;
#6076=FACE_OUTER_BOUND ( 'NONE', #3929, .T. ) ;
#6077=DIRECTION ( 'NONE',  ( -1.000000000000000000, 0.000000000000000000, 0.000000000000000000 ) ) ;
#6078=VECTOR ( 'NONE', #5669, 1000.000000000000000 ) ;
#6081=CARTESIAN_POINT ( 'NONE',  ( 4.789799635567774772, 5.109788315999669095, 8.015886577605016328 ) ) ;
#6086=ORIENTED_EDGE ( 'NONE', *, *, #6204, .T. ) ;
#6091=CARTESIAN_POINT ( 'NONE',  ( 9.020562075079396891E-14, 10.00000000000000000, 729.2499999999977263 ) ) ;
#6098=CIRCLE ( 'NONE', #4394, 4.999999999999993783 ) ;
#6102=DIRECTION ( 'NONE',  ( -0.000000000000000000, -1.000000000000000000, -0.000000000000000000 ) ) ;
#6103=CARTESIAN_POINT ( 'NONE',  ( -52.00000000000006395, 7.999999999999996447, 11.99999999999998934 ) ) ;
#6113=ORIENTED_EDGE ( 'NONE', *, *, #7764, .T. ) ;
#6122=ORIENTED_EDGE ( 'NONE', *, *, #3595, .T. ) ;
#6123=DIRECTION ( 'NONE',  ( -0.000000000000000000, -0.000000000000000000, 1.000000000000000000 ) ) ;
#6134=DIRECTION ( 'NONE',  ( 0.000000000000000000, 0.000000000000000000, -1.000000000000000000 ) ) ;
#6137=ORIENTED_EDGE ( 'NONE', *, *, #5876, .T. ) ;
#6150=CARTESIAN_POINT ( 'NONE',  ( -52.00000000000006395, 7.999999999999996447, 11.99999999999998934 ) ) ;
#6192=CARTESIAN_POINT ( 'NONE',  ( 57.99999999999999289, 7.999999999999996447, 19.99999999999998934 ) ) ;
#6204=EDGE_CURVE ( 'NONE', #6473, #6416, #6356, .T. ) ;
#6231=VECTOR ( 'NONE', #6317, 1000.000000000000000 ) ;
#6244=DIRECTION ( 'NONE',  ( -0.000000000000000000, -0.000000000000000000, 1.000000000000000000 ) ) ;
#6255=EDGE_CURVE ( 'NONE', #4814, #2960, #2399, .T. ) ;
#6258=ORIENTED_EDGE ( 'NONE', *, *, #2561, .T. ) ;
#6260=LINE ( 'NONE', #3107, #5549 ) ;
#6272=CARTESIAN_POINT ( 'NONE',  ( 57.99999999999999289, -8.000000000000001776, 19.99999999999998224 ) ) ;
#6277=ORIENTED_EDGE ( 'NONE', *, *, #3146, .T. ) ;
#6291=LINE ( 'NONE', #5144, #5434 ) ;
#6300=EDGE_LOOP ( 'NONE', ( #1059, #2153, #7462, #1748 ) ) ;
#6305=LINE ( 'NONE', #1280, #6366 ) ;
#6312=FACE_BOUND ( 'NONE', #4652, .T. ) ;
#6317=DIRECTION ( 'NONE',  ( -0.000000000000000000, -1.000000000000000000, -0.000000000000000000 ) ) ;
#6320=ORIENTED_EDGE ( 'NONE', *, *, #398, .T. ) ;
#6326=EDGE_CURVE ( 'NONE', #580, #8077, #7384, .T. ) ;
#6356=CIRCLE ( 'NONE', #6741, 4.999999999999993783 ) ;
#6365=ORIENTED_EDGE ( 'NONE', *, *, #797, .F. ) ;
#6366=VECTOR ( 'NONE', #1743, 1000.000000000000000 ) ;
#6368=ORIENTED_EDGE ( 'NONE', *, *, #5553, .F. ) ;
#6379=ORIENTED_EDGE ( 'NONE', *, *, #5759, .T. ) ;
#6389=DIRECTION ( 'NONE',  ( -0.000000000000000000, -0.000000000000000000, -1.000000000000000000 ) ) ;
#6392=DIRECTION ( 'NONE',  ( 0.000000000000000000, 0.000000000000000000, 1.000000000000000000 ) ) ;
#6414=ORIENTED_EDGE ( 'NONE', *, *, #5876, .F. ) ;
#6415=EDGE_CURVE ( 'NONE', #1461, #6062, #4560, .T. ) ;
#6416=VERTEX_POINT ( 'NONE', #2324 ) ;
#6417=ORIENTED_EDGE ( 'NONE', *, *, #5235, .F. ) ;
#6432=LINE ( 'NONE', #4604, #3569 ) ;
#6434=DIRECTION ( 'NONE',  ( 1.000000000000000000, 0.000000000000000000, 0.000000000000000000 ) ) ;
#6446=ORIENTED_EDGE ( 'NONE', *, *, #4785, .T. ) ;
#6454=DIRECTION ( 'NONE',  ( 1.000000000000000000, 0.000000000000000000, 0.000000000000000000 ) ) ;
#6455=ADVANCED_FACE ( 'NONE', ( #6680 ), #4857, .F. ) ;
#6459=FACE_OUTER_BOUND ( 'NONE', #895, .T. ) ;
#6473=VERTEX_POINT ( 'NONE', #3617 ) ;
#6479=VECTOR ( 'NONE', #4942, 1000.000000000000000 ) ;
#6481=AXIS2_PLACEMENT_3D ( 'NONE', #7454, #466, #5595 ) ;
#6485=B_SPLINE_CURVE_WITH_KNOTS ( 'NONE', 3,
 ( #5426, #7947, #2266, #4677, #1518, #4054, #4343, #1685, #4395, #3639, #427, #6829, #6081, #7986, #470, #6873, #1865, #3005, #1817, #4885, #2474, #2343, #7457, #8155, #1774 ),
 .UNSPECIFIED., .F., .F.,
 ( 4, 2, 2, 1, 2, 2, 2, 2, 2, 2, 2, 2, 4 ),
 ( 0.02188532927265061934, 0.02325358088725200043, 0.02393770669455269270, 0.02462183250185338151, 0.02530595830915407379, 0.02599008411645476260, 0.02735833573105614369, 0.02804246153835683597, 0.02872658734565752478, 0.03009483896025890587, 0.03077896476755959815, 0.03146309057486028349, 0.03283134218946166805 ),
 .UNSPECIFIED. ) ;
#6511=ORIENTED_EDGE ( 'NONE', *, *, #3875, .T. ) ;
#6516=EDGE_CURVE ( 'NONE', #2553, #3093, #3031, .T. ) ;
#6522=ORIENTED_EDGE ( 'NONE', *, *, #329, .T. ) ;
#6531=CARTESIAN_POINT ( 'NONE',  ( 52.00000000000000000, 7.999999999999996447, 11.99999999999998934 ) ) ;
#6550=ORIENTED_EDGE ( 'NONE', *, *, #2178, .T. ) ;
#6553=DIRECTION ( 'NONE',  ( 1.000000000000000000, 0.000000000000000000, -0.000000000000000000 ) ) ;
#6565=CARTESIAN_POINT ( 'NONE',  ( 55.00000000000000000, 10.00000000000000000, 17.64999999999999858 ) ) ;
#6579=DIRECTION ( 'NONE',  ( 1.000000000000000000, -0.000000000000000000, 0.000000000000000000 ) ) ;
#6580=DIRECTION ( 'NONE',  ( 0.000000000000000000, 0.000000000000000000, 1.000000000000000000 ) ) ;
#6586=CIRCLE ( 'NONE', #3550, 2.149999999999992362 ) ;
#6587=DIRECTION ( 'NONE',  ( -0.000000000000000000, -0.000000000000000000, -1.000000000000000000 ) ) ;
#6601=VECTOR ( 'NONE', #6026, 1000.000000000000000 ) ;
#6614=AXIS2_PLACEMENT_3D ( 'NONE', #2688, #2534, #6392 ) ;
#6615=SURFACE_STYLE_FILL_AREA ( #1551 ) ;
#6625=LINE ( 'NONE', #2768, #1700 ) ;
#6630=EDGE_CURVE ( 'NONE', #471, #5793, #6432, .T. ) ;
#6634=ORIENTED_EDGE ( 'NONE', *, *, #5351, .T. ) ;
#6636=AXIS2_PLACEMENT_3D ( 'NONE', #3902, #5736, #7006 ) ;
#6647=VERTEX_POINT ( 'NONE', #698 ) ;
#6650=CARTESIAN_POINT ( 'NONE',  ( 9.020562060468115204E-14, -7.000000000000000000, 7.999999999999977796 ) ) ;
#6662=DIRECTION ( 'NONE',  ( 1.000000000000000000, 0.000000000000000000, 0.000000000000000000 ) ) ;
#6671=CARTESIAN_POINT ( 'NONE',  ( -54.99999999999990052, 10.00000000000000000, 15.49999999999877254 ) ) ;
#6680=FACE_OUTER_BOUND ( 'NONE', #783, .T. ) ;
#6682=CARTESIAN_POINT ( 'NONE',  ( -6.063573224773413095, 3.505086101364692563, 8.025480671672065469 ) ) ;
#6685=ADVANCED_FACE ( 'NONE', ( #67 ), #2006, .F. ) ;
#6724=DIRECTION ( 'NONE',  ( 0.000000000000000000, 0.000000000000000000, 1.000000000000000000 ) ) ;
#6729=EDGE_CURVE ( 'NONE', #7794, #1727, #1611, .T. ) ;
#6731=DIRECTION ( 'NONE',  ( 1.000000000000000000, 0.000000000000000000, 0.000000000000000000 ) ) ;
#6741=AXIS2_PLACEMENT_3D ( 'NONE', #3065, #8082, #3011 ) ;
#6745=FILL_AREA_STYLE_COLOUR ( '', #3903 ) ;
#6765=DIRECTION ( 'NONE',  ( -0.000000000000000000, 1.000000000000000000, -0.000000000000000000 ) ) ;
#6768=CARTESIAN_POINT ( 'NONE',  ( -3.505070609393837522, 6.076439379008851560, 8.008416788275647846 ) ) ;
#6769=AXIS2_PLACEMENT_3D ( 'NONE', #4516, #5680, #3775 ) ;
#6772=AXIS2_PLACEMENT_3D ( 'NONE', #1242, #6928, #3826 ) ;
#6774=ORIENTED_EDGE ( 'NONE', *, *, #2178, .F. ) ;
#6775=EDGE_CURVE ( 'NONE', #7382, #5247, #4490, .T. ) ;
#6786=CYLINDRICAL_SURFACE ( 'NONE', #3977, 2.149999999999995470 ) ;
#6797=DIRECTION ( 'NONE',  ( 1.000000000000000000, 0.000000000000000000, -0.000000000000000000 ) ) ;
#6804=DIRECTION ( 'NONE',  ( -1.000000000000000000, 0.000000000000000000, 0.000000000000000000 ) ) ;
#6807=CARTESIAN_POINT ( 'NONE',  ( -1.588057467863390526, 6.821288780608425917, 8.001713687856982560 ) ) ;
#6817=CARTESIAN_POINT ( 'NONE',  ( 9.020562075079396891E-14, 10.00000000000000000, 729.2499999999977263 ) ) ;
#6825=LINE ( 'NONE', #4297, #5427 ) ;
#6828=CARTESIAN_POINT ( 'NONE',  ( -6.632365264926793458, -2.250456567307095757, 8.030492030296132455 ) ) ;
#6829=CARTESIAN_POINT ( 'NONE',  ( 5.273939683826339930, 4.625367979329794821, 8.019210142024537191 ) ) ;
#6851=ORIENTED_EDGE ( 'NONE', *, *, #4013, .T. ) ;
#6852=ORIENTED_EDGE ( 'NONE', *, *, #6255, .F. ) ;
#6865=EDGE_CURVE ( 'NONE', #2944, #3913, #6260, .T. ) ;
#6873=CARTESIAN_POINT ( 'NONE',  ( 4.077904861489376032, 5.694132991774995212, 8.011503056869331729 ) ) ;
#6876=VERTEX_POINT ( 'NONE', #8124 ) ;
#6906=CARTESIAN_POINT ( 'NONE',  ( 52.00000000000000000, -8.000000000000003553, 11.99999999999998934 ) ) ;
#6917=EDGE_LOOP ( 'NONE', ( #2429, #5074, #2219, #1749 ) ) ;
#6918=MANIFOLD_SOLID_BREP ( 'M4 Clearance Hole1', #7797 ) ;
#6921=CARTESIAN_POINT ( 'NONE',  ( -54.99999999999990052, -8.000000000000001776, 15.49999999999877254 ) ) ;
#6928=DIRECTION ( 'NONE',  ( 0.000000000000000000, -1.000000000000000000, 0.000000000000000000 ) ) ;
#6931=EDGE_CURVE ( 'NONE', #4508, #2164, #756, .T. ) ;
#6933=DIRECTION ( 'NONE',  ( 1.000000000000000000, 0.000000000000000000, 0.000000000000000000 ) ) ;
#6947=CARTESIAN_POINT ( 'NONE',  ( -58.00000000000006395, 7.999999999999996447, 11.99999999999998934 ) ) ;
#6951=VERTEX_POINT ( 'NONE', #5732 ) ;
#6965=CARTESIAN_POINT ( 'NONE',  ( -52.00000000000006395, 7.999999999999996447, 11.99999999999998934 ) ) ;
#6967=CARTESIAN_POINT ( 'NONE',  ( 0.000000000000000000, 0.000000000000000000, 0.000000000000000000 ) ) ;
#6970=ADVANCED_FACE ( 'NONE', ( #7002 ), #1949, .F. ) ;
#6972=CARTESIAN_POINT ( 'NONE',  ( -52.00000000000006395, -8.000000000000003553, 11.99999999999998934 ) ) ;
#6981=EDGE_LOOP ( 'NONE', ( #1308, #7685, #6852, #6122 ) ) ;
#6995=EDGE_CURVE ( 'NONE', #5386, #3008, #7713, .T. ) ;
#7002=FACE_OUTER_BOUND ( 'NONE', #3367, .T. ) ;
#7006=DIRECTION ( 'NONE',  ( 0.000000000000000000, 0.000000000000000000, 1.000000000000000000 ) ) ;
#7008=EDGE_CURVE ( 'NONE', #5475, #7622, #5848, .T. ) ;
#7033=VECTOR ( 'NONE', #1644, 1000.000000000000000 ) ;
#7039=CIRCLE ( 'NONE', #2010, 2.149999999999992362 ) ;
#7044=CARTESIAN_POINT ( 'NONE',  ( -2.252029883699507629, -6.631804555459141604, 8.003482568582050760 ) ) ;
#7053=ORIENTED_EDGE ( 'NONE', *, *, #3836, .T. ) ;
#7072=ORIENTED_EDGE ( 'NONE', *, *, #5660, .F. ) ;
#7083=CARTESIAN_POINT ( 'NONE',  ( -2.650000000000006128, 3.245314017740489413E-16, 20.00000000000000355 ) ) ;
#7085=DIRECTION ( 'NONE',  ( 0.000000000000000000, 0.000000000000000000, -1.000000000000000000 ) ) ;
#7094=DIRECTION ( 'NONE',  ( 1.000000000000000000, 0.000000000000000000, 0.000000000000000000 ) ) ;
#7109=ORIENTED_EDGE ( 'NONE', *, *, #3538, .F. ) ;
#7128=LINE ( 'NONE', #2692, #1400 ) ;
#7131=PLANE ( 'NONE',  #8197 ) ;
#7132=LINE ( 'NONE', #4646, #99 ) ;
#7137=VECTOR ( 'NONE', #2161, 1000.000000000000000 ) ;
#7143=FACE_OUTER_BOUND ( 'NONE', #7639, .T. ) ;
#7149=ADVANCED_FACE ( 'NONE', ( #2213 ), #967, .F. ) ;
#7152=ORIENTED_EDGE ( 'NONE', *, *, #6729, .F. ) ;
#7159=EDGE_CURVE ( 'NONE', #2122, #2164, #2879, .T. ) ;
#7172=DIRECTION ( 'NONE',  ( 0.000000000000000000, 0.000000000000000000, -1.000000000000000000 ) ) ;
#7173=CARTESIAN_POINT ( 'NONE',  ( -54.99999999999990052, 10.00000000000000000, 17.64999999999876934 ) ) ;
#7177=DIRECTION ( 'NONE',  ( -0.000000000000000000, 1.000000000000000000, -0.000000000000000000 ) ) ;
#7178=ORIENTED_EDGE ( 'NONE', *, *, #4785, .F. ) ;
#7213=LINE ( 'NONE', #1615, #4914 ) ;
#7221=CARTESIAN_POINT ( 'NONE',  ( -52.00000000000006395, -8.000000000000003553, 19.99999999999998934 ) ) ;
#7251=EDGE_LOOP ( 'NONE', ( #240, #6774, #6379, #533 ) ) ;
#7261=CARTESIAN_POINT ( 'NONE',  ( -4.625276930412667298, 5.274027880968991333, 8.014758447098458305 ) ) ;
#7277=VECTOR ( 'NONE', #3453, 1000.000000000000000 ) ;
#7305=ORIENTED_EDGE ( 'NONE', *, *, #400, .F. ) ;
#7311=CARTESIAN_POINT ( 'NONE',  ( -6.954674599839328231, 0.9195257330843505938, 8.033525432897004492 ) ) ;
#7316=ORIENTED_EDGE ( 'NONE', *, *, #4937, .F. ) ;
#7318=CARTESIAN_POINT ( 'NONE',  ( 4.622735087487665595, -5.276717374392886128, 8.014740495741826010 ) ) ;
#7327=CARTESIAN_POINT ( 'NONE',  ( -6.554102889824980238, -2.469088713791839140, 8.029774298059875193 ) ) ;
#7342=ORIENTED_EDGE ( 'NONE', *, *, #1009, .F. ) ;
#7345=CARTESIAN_POINT ( 'NONE',  ( 4.999999999999990230, 0.000000000000000000, 20.00000000000000355 ) ) ;
#7349=CARTESIAN_POINT ( 'NONE',  ( -6.377569469000553326, 2.894565604611681664, 8.028191719259677228 ) ) ;
#7350=CARTESIAN_POINT ( 'NONE',  ( 57.99999999999999289, 7.999999999999996447, 11.99999999999998934 ) ) ;
#7363=( LENGTH_UNIT ( ) NAMED_UNIT ( * ) SI_UNIT ( .MILLI., .METRE. ) );
#7372=CARTESIAN_POINT ( 'NONE',  ( 60.00000000000014211, 10.00000000000000000, 10.50000000000006395 ) ) ;
#7375=DIRECTION ( 'NONE',  ( 0.000000000000000000, 0.000000000000000000, 1.000000000000000000 ) ) ;
#7377=AXIS2_PLACEMENT_3D ( 'NONE', #1337, #5888, #35 ) ;
#7382=VERTEX_POINT ( 'NONE', #2871 ) ;
#7384=LINE ( 'NONE', #6103, #2369 ) ;
#7390=CIRCLE ( 'NONE', #5415, 2.149999999999995470 ) ;
#7406=FACE_BOUND ( 'NONE', #2456, .T. ) ;
#7410=EDGE_CURVE ( 'NONE', #6416, #6473, #6098, .T. ) ;
#7412=AXIS2_PLACEMENT_3D ( 'NONE', #2284, #6055, #357 ) ;
#7413=CARTESIAN_POINT ( 'NONE',  ( 0.000000000000000000, 0.000000000000000000, 20.00000000000000355 ) ) ;
#7416=EDGE_LOOP ( 'NONE', ( #5133, #3371 ) ) ;
#7426=PRODUCT_DEFINITION_SHAPE ( 'NONE', 'NONE',  #5748 ) ;
#7427=ORIENTED_EDGE ( 'NONE', *, *, #6775, .T. ) ;
#7434=EDGE_CURVE ( 'NONE', #4369, #5370, #875, .T. ) ;
#7446=CARTESIAN_POINT ( 'NONE',  ( 9.020562075079396891E-14, -10.00000000000000000, 729.2499999999977263 ) ) ;
#7454=CARTESIAN_POINT ( 'NONE',  ( 9.020562075079396891E-14, -10.00000000000000000, 729.2499999999977263 ) ) ;
#7457=CARTESIAN_POINT ( 'NONE',  ( 0.9164596775857979383, 6.954740550032190605, 8.000443323644105931 ) ) ;
#7462=ORIENTED_EDGE ( 'NONE', *, *, #2444, .T. ) ;
#7466=DIRECTION ( 'NONE',  ( 0.000000000000000000, 0.000000000000000000, 1.000000000000000000 ) ) ;
#7471=VERTEX_POINT ( 'NONE', #369 ) ;
#7495=ORIENTED_EDGE ( 'NONE', *, *, #5351, .F. ) ;
#7496=PLANE ( 'NONE',  #6481 ) ;
#7502=ORIENTED_EDGE ( 'NONE', *, *, #4034, .F. ) ;
#7505=DIRECTION ( 'NONE',  ( -0.000000000000000000, -0.000000000000000000, 1.000000000000000000 ) ) ;
#7512=DIRECTION ( 'NONE',  ( 0.000000000000000000, 1.000000000000000000, -0.000000000000000000 ) ) ;
#7523=ORIENTED_EDGE ( 'NONE', *, *, #7565, .T. ) ;
#7526=CARTESIAN_POINT ( 'NONE',  ( 2.649999999999991918, 0.000000000000000000, 1.040834085586084257E-14 ) ) ;
#7532=VERTEX_POINT ( 'NONE', #7526 ) ;
#7551=CARTESIAN_POINT ( 'NONE',  ( -58.00000000000006395, 7.999999999999996447, 11.99999999999998934 ) ) ;
#7554=DIRECTION ( 'NONE',  ( -0.000000000000000000, -0.000000000000000000, 1.000000000000000000 ) ) ;
#7556=ORIENTED_EDGE ( 'NONE', *, *, #3057, .T. ) ;
#7558=DIRECTION ( 'NONE',  ( 1.000000000000000000, 0.000000000000000000, 0.000000000000000000 ) ) ;
#7565=EDGE_CURVE ( 'NONE', #3093, #2445, #3668, .T. ) ;
#7574=VERTEX_POINT ( 'NONE', #4920 ) ;
#7579=AXIS2_PLACEMENT_3D ( 'NONE', #5115, #4021, #759 ) ;
#7597=SURFACE_STYLE_FILL_AREA ( #431 ) ;
#7601=DIRECTION ( 'NONE',  ( 0.000000000000000000, 0.000000000000000000, 1.000000000000000000 ) ) ;
#7610=VERTEX_POINT ( 'NONE', #6192 ) ;
#7622=VERTEX_POINT ( 'NONE', #3761 ) ;
#7631=VERTEX_POINT ( 'NONE', #1389 ) ;
#7637=CYLINDRICAL_SURFACE ( 'NONE', #6636, 2.149999999999995470 ) ;
#7639=EDGE_LOOP ( 'NONE', ( #3262, #6320, #984, #7053 ) ) ;
#7648=ORIENTED_EDGE ( 'NONE', *, *, #329, .F. ) ;
#7653=DIRECTION ( 'NONE',  ( -0.000000000000000000, -1.000000000000000000, -0.000000000000000000 ) ) ;
#7672=CARTESIAN_POINT ( 'NONE',  ( 52.00000000000000000, 7.999999999999996447, 11.99999999999998934 ) ) ;
#7685=ORIENTED_EDGE ( 'NONE', *, *, #4147, .F. ) ;
#7686=EDGE_CURVE ( 'NONE', #7574, #2944, #2505, .T. ) ;
#7687=AXIS2_PLACEMENT_3D ( 'NONE', #1813, #8151, #5509 ) ;
#7693=ORIENTED_EDGE ( 'NONE', *, *, #1846, .F. ) ;
#7696=DIRECTION ( 'NONE',  ( 0.000000000000000000, 0.000000000000000000, 1.000000000000000000 ) ) ;
#7701=ORIENTED_EDGE ( 'NONE', *, *, #1009, .T. ) ;
#7709=CARTESIAN_POINT ( 'NONE',  ( -3.698018259095727789, -5.947912380466928717, 8.009454966680493726 ) ) ;
#7713=LINE ( 'NONE', #2572, #661 ) ;
#7733=EDGE_CURVE ( 'NONE', #8077, #2944, #4421, .T. ) ;
#7747=DIRECTION ( 'NONE',  ( 0.000000000000000000, 0.000000000000000000, 1.000000000000000000 ) ) ;
#7748=FACE_OUTER_BOUND ( 'NONE', #364, .T. ) ;
#7749=FACE_OUTER_BOUND ( 'NONE', #5494, .T. ) ;
#7764=EDGE_CURVE ( 'NONE', #3149, #2847, #7039, .T. ) ;
#7787=AXIS2_PLACEMENT_3D ( 'NONE', #639, #1945, #1863 ) ;
#7788=CARTESIAN_POINT ( 'NONE',  ( 57.99999999999999289, -8.000000000000003553, 11.99999999999998934 ) ) ;
#7790=ORIENTED_EDGE ( 'NONE', *, *, #2561, .F. ) ;
#7794=VERTEX_POINT ( 'NONE', #3480 ) ;
#7797=CLOSED_SHELL ( 'NONE', ( #963, #6970, #4818, #2151, #1585, #2073, #7882, #2958, #1315, #1008, #5375, #4452, #7819, #2877, #4789, #2682, #7149, #1999, #5902, #836, #5139, #4274, #4276, #6685, #5526, #2232, #3200, #454, #3406, #8145, #4850, #6455, #2042 ) ) ;
#7799=AXIS2_PLACEMENT_3D ( 'NONE', #2503, #7653, #710 ) ;
#7807=AXIS2_PLACEMENT_3D ( 'NONE', #6091, #4103, #8032 ) ;
#7815=AXIS2_PLACEMENT_3D ( 'NONE', #2030, #1320, #7747 ) ;
#7819=ADVANCED_FACE ( 'NONE', ( #4808 ), #4182, .F. ) ;
#7825=( NAMED_UNIT ( * ) PLANE_ANGLE_UNIT ( ) SI_UNIT ( $, .RADIAN. ) );
#7844=DIRECTION ( 'NONE',  ( -0.000000000000000000, -0.000000000000000000, 1.000000000000000000 ) ) ;
#7858=DIRECTION ( 'NONE',  ( 0.000000000000000000, 1.000000000000000000, -0.000000000000000000 ) ) ;
#7863=DIRECTION ( 'NONE',  ( 0.000000000000000000, 0.000000000000000000, 1.000000000000000000 ) ) ;
#7873=VERTEX_POINT ( 'NONE', #1565 ) ;
#7874=DIRECTION ( 'NONE',  ( -1.000000000000000000, 0.000000000000000000, 0.000000000000000000 ) ) ;
#7882=ADVANCED_FACE ( 'NONE', ( #4140 ), #6004, .T. ) ;
#7911=ORIENTED_EDGE ( 'NONE', *, *, #7434, .F. ) ;
#7914=CARTESIAN_POINT ( 'NONE',  ( 57.99999999999999289, -8.000000000000003553, 19.99999999999998934 ) ) ;
#7918=CARTESIAN_POINT ( 'NONE',  ( -6.773732078532765932, 1.824713701299700563, 8.031803308098282912 ) ) ;
#7926=EDGE_LOOP ( 'NONE', ( #492, #908, #1503, #630 ) ) ;
#7947=CARTESIAN_POINT ( 'NONE',  ( 7.000000000000000000, 0.4570009800896051022, 8.033969604113655905 ) ) ;
#7954=CARTESIAN_POINT ( 'NONE',  ( -58.00000000000006395, 7.999999999999996447, 19.99999999999998934 ) ) ;
#7959=DIRECTION ( 'NONE',  ( -1.000000000000000000, 0.000000000000000000, 0.000000000000000000 ) ) ;
#7973=ORIENTED_EDGE ( 'NONE', *, *, #2709, .T. ) ;
#7986=CARTESIAN_POINT ( 'NONE',  ( 4.620169681576417275, 5.263757874614205079, 8.014776054765157198 ) ) ;
#8004=CARTESIAN_POINT ( 'NONE',  ( -3.103177678536665596, 6.291349734783570291, 8.006551011514465799 ) ) ;
#8026=FACE_BOUND ( 'NONE', #4612, .T. ) ;
#8032=DIRECTION ( 'NONE',  ( 0.000000000000000000, 0.000000000000000000, -1.000000000000000000 ) ) ;
#8033=PLANE ( 'NONE',  #4775 ) ;
#8034=CARTESIAN_POINT ( 'NONE',  ( -7.562723597472470821E-15, -3.402841154990142473E-15, 11.99999999999998934 ) ) ;
#8037=CIRCLE ( 'NONE', #1682, 2.149999999999999023 ) ;
#8046=EDGE_CURVE ( 'NONE', #2461, #7794, #6305, .T. ) ;
#8047=AXIS2_PLACEMENT_3D ( 'NONE', #6921, #1905, #5146 ) ;
#8051=ORIENTED_EDGE ( 'NONE', *, *, #1723, .F. ) ;
#8052=EDGE_LOOP ( 'NONE', ( #1958, #2571, #323, #5132 ) ) ;
#8055=DIRECTION ( 'NONE',  ( 0.000000000000000000, 0.000000000000000000, -1.000000000000000000 ) ) ;
#8067=DIRECTION ( 'NONE',  ( -0.000000000000000000, 1.000000000000000000, -0.000000000000000000 ) ) ;
#8070=CARTESIAN_POINT ( 'NONE',  ( -6.954591388923755169, -0.9174941424614954100, 8.033524818493585684 ) ) ;
#8077=VERTEX_POINT ( 'NONE', #8161 ) ;
#8078=AXIS2_PLACEMENT_3D ( 'NONE', #2352, #1107, #7375 ) ;
#8080=CARTESIAN_POINT ( 'NONE',  ( 55.00000000000000000, -8.000000000000001776, 15.50000000000000355 ) ) ;
#8082=DIRECTION ( 'NONE',  ( -0.000000000000000000, -0.000000000000000000, 1.000000000000000000 ) ) ;
#8088=CARTESIAN_POINT ( 'NONE',  ( 55.00000000000000000, -10.00000000000000000, 15.50000000000000355 ) ) ;
#8092=ORIENTED_EDGE ( 'NONE', *, *, #6865, .F. ) ;
#8119=EDGE_CURVE ( 'NONE', #2900, #5567, #239, .T. ) ;
#8122=ORIENTED_EDGE ( 'NONE', *, *, #7764, .F. ) ;
#8124=CARTESIAN_POINT ( 'NONE',  ( -60.00000000000000000, 10.00000000000000000, 10.50000000000000000 ) ) ;
#8127=CARTESIAN_POINT ( 'NONE',  ( 7.000000000000000000, 8.572527594031473190E-16, 0.000000000000000000 ) ) ;
#8135=DIRECTION ( 'NONE',  ( 0.000000000000000000, -0.000000000000000000, -1.000000000000000000 ) ) ;
#8136=CARTESIAN_POINT ( 'NONE',  ( -60.00000000000000000, 10.00000000000000000, 20.00000000000000355 ) ) ;
#8145=ADVANCED_FACE ( 'NONE', ( #98 ), #1482, .F. ) ;
#8151=DIRECTION ( 'NONE',  ( -0.000000000000000000, -0.000000000000000000, 1.000000000000000000 ) ) ;
#8154=CARTESIAN_POINT ( 'NONE',  ( -5.566961118109779783, -4.268296125650788753, 8.021439803987641781 ) ) ;
#8155=CARTESIAN_POINT ( 'NONE',  ( 0.4618352976297687151, 6.999999999999993783, 8.000000000000024869 ) ) ;
#8159=EDGE_LOOP ( 'NONE', ( #4678, #1022, #5832, #5792 ) ) ;
#8161=CARTESIAN_POINT ( 'NONE',  ( -58.00000000000006395, 7.999999999999996447, 11.99999999999998934 ) ) ;
#8163=LINE ( 'NONE', #3742, #2913 ) ;
#8165=DIRECTION ( 'NONE',  ( -0.000000000000000000, 1.000000000000000000, -0.000000000000000000 ) ) ;
#8170=FACE_OUTER_BOUND ( 'NONE', #882, .T. ) ;
#8176=ORIENTED_EDGE ( 'NONE', *, *, #179, .F. ) ;
#8178=ORIENTED_EDGE ( 'NONE', *, *, #8119, .T. ) ;
#8183=DIRECTION ( 'NONE',  ( 1.000000000000000000, 0.000000000000000000, 0.000000000000000000 ) ) ;
#8191=CYLINDRICAL_SURFACE ( 'NONE', #7787, 2.650000000000002576 ) ;
#8194=CARTESIAN_POINT ( 'NONE',  ( 9.020562060468115204E-14, -7.000000000000000000, 7.999999999999977796 ) ) ;
#8197=AXIS2_PLACEMENT_3D ( 'NONE', #7788, #5208, #5316 ) ;
ENDSEC;
END-ISO-10303-21;
